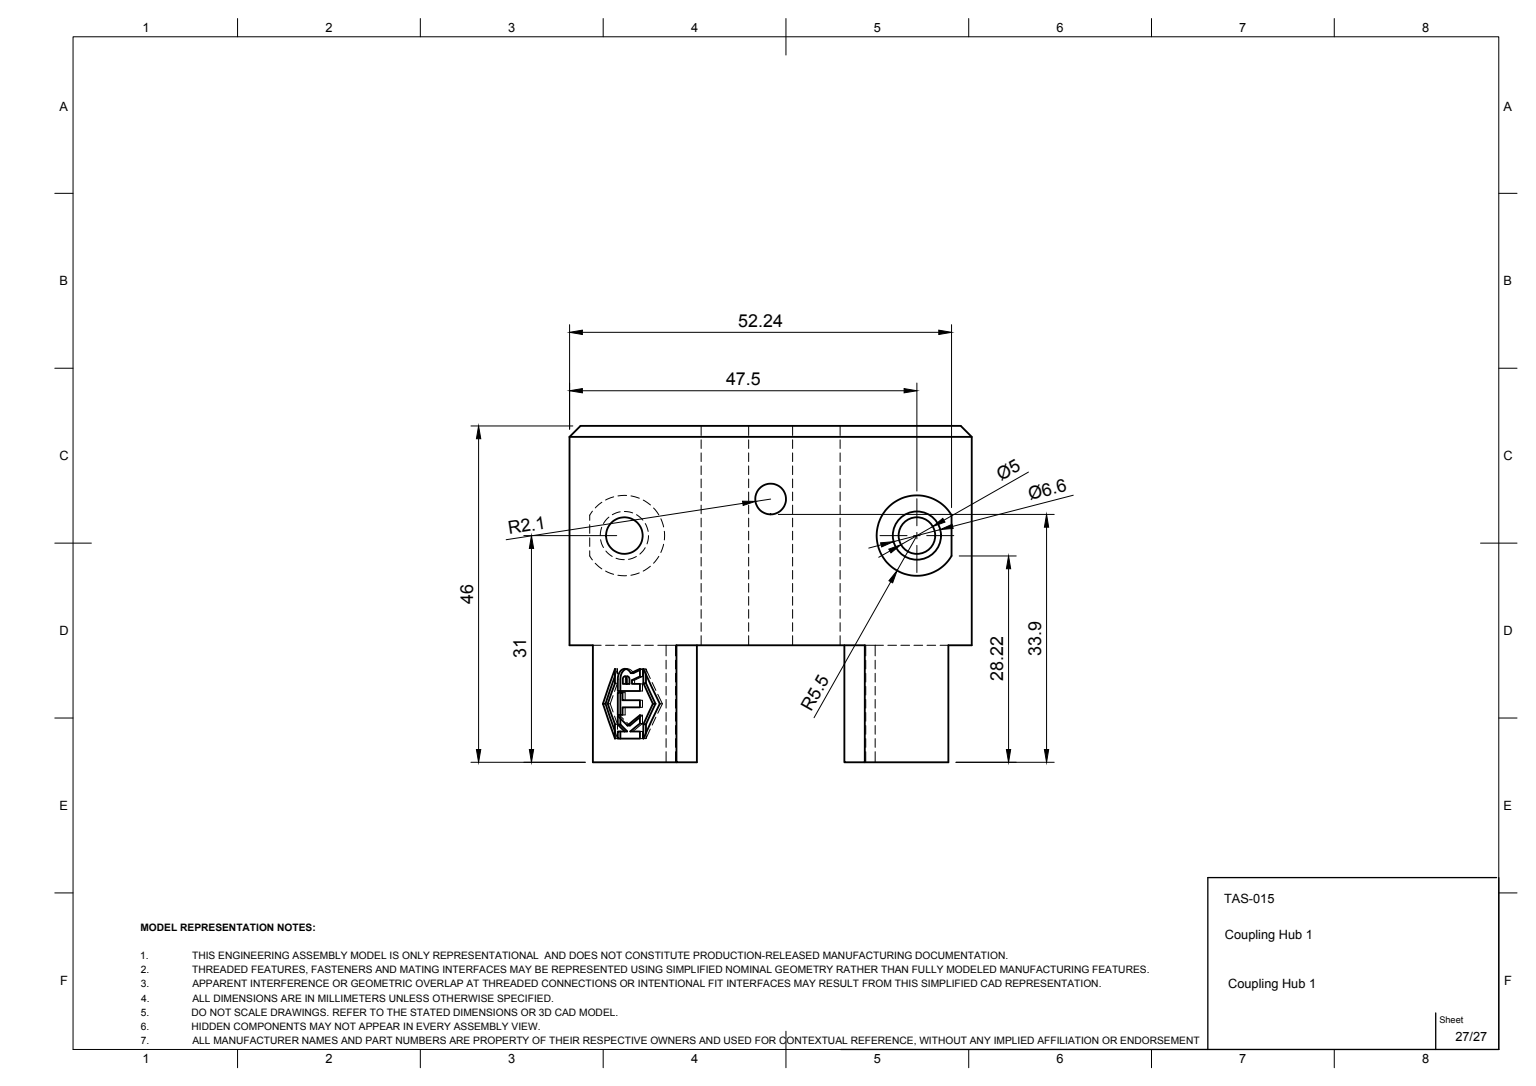
ISO-10303-21;
HEADER;
/* Generated by software containing ST-Developer
 * from STEP Tools, Inc. (www.steptools.com) 
 */

FILE_DESCRIPTION(
/* description */ ('STEP AP214'),
/* implementation_level */ '2;1');

FILE_NAME(
/* name */ 'Coupling Hub 1.step',
/* time_stamp */ '2026-11-15T14:49:54-08:00',
/* author */ (''),
/* organization */ (''),
/* preprocessor_version */ 'ST-DEVELOPER v20.2',
/* originating_system */ 'Autodesk Translation Framework v15.17.0.0',
/* authorisation */ '');

FILE_SCHEMA (('AUTOMOTIVE_DESIGN { 1 0 10303 214 3 1 1 }'));
ENDSEC;

DATA;
#10=MECHANICAL_DESIGN_GEOMETRIC_PRESENTATION_REPRESENTATION('',(#1124,#1125),#66721);
#389=B_SPLINE_CURVE_WITH_KNOTS('',3,(#65265,#65266,#65267,#65268,#65269,
#65270,#65271,#65272,#65273,#65274,#65275,#65276,#65277,#65278,#65279,#65280,
#65281,#65282),.UNSPECIFIED.,.F.,.F.,(4,2,2,2,2,2,2,2,4),(0.567634871261072,
0.624046753013484,0.757510403489333,0.849653931020164,0.941797458550995,
1.03394098608183,1.12608451361266,1.25954816408851,1.39301181456436),
 .UNSPECIFIED.);
#390=B_SPLINE_CURVE_WITH_KNOTS('',3,(#65283,#65284,#65285,#65286,#65287,
#65288,#65289,#65290,#65291,#65292,#65293,#65294,#65295,#65296,#65297,#65298,
#65299,#65300,#65301,#65302,#65303,#65304,#65305,#65306,#65307),
 .UNSPECIFIED.,.F.,.F.,(4,2,2,2,2,3,2,2,2,2,2,4),(1.39301181456436,1.54288207354147,
1.69275233251858,1.78817362481028,1.83588427095614,1.88359491710199,1.93130556324784,
1.97901620939369,2.0744375016854,2.22430776066251,2.37417801963962,2.45122978836306),
 .UNSPECIFIED.);
#391=B_SPLINE_CURVE_WITH_KNOTS('',3,(#65311,#65312,#65313,#65314,#65315,
#65316,#65317,#65318,#65319,#65320,#65321,#65322,#65323,#65324,#65325,#65326,
#65327,#65328,#65329,#65330,#65331,#65332,#65333,#65334,#65335,#65336,#65337,
#65338,#65339,#65340),.UNSPECIFIED.,.F.,.F.,(4,2,2,2,2,2,2,2,2,2,2,2,2,
2,4),(-3.98325608641923,-3.86919217466994,-3.49972652064847,-3.130260866627,
-2.85088285941104,-2.57150485219509,-2.36940240570498,-2.16729995921487,
-1.96519751272476,-1.76309506623465,-1.4837170590187,-1.20433905180275,
-0.834873397781281,-0.465407743759808,-0.351343832010516),.UNSPECIFIED.);
#392=B_SPLINE_CURVE_WITH_KNOTS('',3,(#65376,#65377,#65378,#65379,#65380,
#65381,#65382,#65383,#65384,#65385,#65386,#65387,#65388,#65389,#65390,#65391,
#65392,#65393,#65394,#65395,#65396,#65397,#65398,#65399,#65400,#65401,#65402,
#65403,#65404,#65405),.UNSPECIFIED.,.F.,.F.,(4,2,2,2,2,2,2,2,2,2,2,2,2,
2,4),(-3.98325608641923,-3.86919217466994,-3.49972652064847,-3.130260866627,
-2.85088285941104,-2.57150485219509,-2.36940240570498,-2.16729995921487,
-1.96519751272476,-1.76309506623465,-1.4837170590187,-1.20433905180275,
-0.834873397781281,-0.465407743759808,-0.351343832010517),.UNSPECIFIED.);
#393=B_SPLINE_CURVE_WITH_KNOTS('',3,(#65422,#65423,#65424,#65425,#65426,
#65427,#65428,#65429,#65430,#65431,#65432,#65433,#65434,#65435,#65436,#65437,
#65438,#65439,#65440,#65441,#65442,#65443,#65444,#65445,#65446,#65447,#65448,
#65449),.UNSPECIFIED.,.F.,.F.,(4,2,2,2,2,2,2,2,2,2,2,2,2,4),(0.490583102537635,
0.624046753013484,0.757510403489333,0.849653931020164,0.941797458550995,
1.03394098608183,1.12608451361266,1.25954816408851,1.39301181456436,1.54288207354147,
1.69275233251858,1.78817362481028,1.83588427095614,1.88359491710199),
 .UNSPECIFIED.);
#394=B_SPLINE_CURVE_WITH_KNOTS('',3,(#65450,#65451,#65452,#65453,#65454,
#65455,#65456,#65457,#65458,#65459,#65460,#65461),.UNSPECIFIED.,.F.,.F.,
(4,2,2,2,2,4),(0.,0.0477106461458525,0.095421292291705,0.19084258458341,
0.340712843560522,0.490583102537635),.UNSPECIFIED.);
#395=B_SPLINE_CURVE_WITH_KNOTS('',3,(#65538,#65539,#65540,#65541,#65542,
#65543,#65544,#65545,#65546,#65547,#65548,#65549,#65550,#65551,#65552,#65553,
#65554,#65555),.UNSPECIFIED.,.F.,.F.,(4,2,2,2,2,2,2,2,4),(0.,0.0151927838523538,
0.0303855677047076,0.0455818431537581,0.0607781186028085,0.0759788205112385,
0.0911795224196684,0.106372746681134,0.1215659709426),.UNSPECIFIED.);
#396=B_SPLINE_CURVE_WITH_KNOTS('',3,(#65565,#65566,#65567,#65568,#65569,
#65570,#65571,#65572,#65573,#65574,#65575,#65576,#65577,#65578,#65579,#65580,
#65581,#65582),.UNSPECIFIED.,.F.,.F.,(4,2,2,2,2,2,2,2,4),(0.316549052084077,
0.395686269484847,0.474823486885617,0.553960795526886,0.633098104168155,
0.712235412809424,0.791372721450693,0.870509938851463,0.949647156252233),
 .UNSPECIFIED.);
#397=B_SPLINE_CURVE_WITH_KNOTS('',3,(#65584,#65585,#65586,#65587,#65588,
#65589,#65590,#65591,#65592,#65593,#65594,#65595,#65596,#65597,#65598,#65599,
#65600,#65601,#65602,#65603,#65604,#65605,#65606,#65607,#65608,#65609,#65610,
#65611,#65612,#65613,#65614,#65615,#65616,#65617,#65618,#65619,#65620,#65621,
#65622,#65623,#65624,#65625,#65626,#65627,#65628,#65629,#65630,#65631,#65632,
#65633,#65634,#65635,#65636,#65637,#65638,#65639,#65640,#65641,#65642,#65643,
#65644),.UNSPECIFIED.,.F.,.F.,(4,3,3,3,3,3,3,3,3,3,3,3,3,3,3,3,3,3,3,3,
4),(0.,0.0530381007183943,0.106881831871485,0.160741064784848,0.214029096098922,
0.25,0.302729149593727,0.356241664754916,0.409762787712598,0.462708186143729,
0.5,0.552255845606725,0.605282211731377,0.658318725202785,0.710788396890028,
0.75,0.802421738286123,0.855626872467919,0.908846463729713,0.961502691971665,
1.),.UNSPECIFIED.);
#398=B_SPLINE_CURVE_WITH_KNOTS('',3,(#65645,#65646,#65647,#65648,#65649,
#65650,#65651,#65652,#65653,#65654),.UNSPECIFIED.,.F.,.F.,(4,2,2,2,4),(0.949647156252233,
1.028784373653,1.10792159105377,1.18705889969504,1.26619620833631),
 .UNSPECIFIED.);
#399=B_SPLINE_CURVE_WITH_KNOTS('',3,(#65695,#65696,#65697,#65698,#65699,
#65700,#65701,#65702,#65703,#65704,#65705,#65706,#65707,#65708,#65709,#65710),
 .UNSPECIFIED.,.F.,.F.,(4,2,2,2,2,2,2,4),(-0.779703847201593,-0.757646703299412,
-0.7035492015768,-0.649451699854188,-0.595298023055894,-0.5411443462576,
-0.487035463795603,-0.432926581333605),.UNSPECIFIED.);
#400=B_SPLINE_CURVE_WITH_KNOTS('',3,(#65933,#65934,#65935,#65936,#65937,
#65938,#65939,#65940,#65941,#65942,#65943,#65944,#65945,#65946,#65947,#65948),
 .UNSPECIFIED.,.F.,.F.,(4,2,2,2,2,2,2,4),(0.432932407296797,0.487041759940904,
0.541151112585012,0.595306935250484,0.649462757915956,0.703560301016107,
0.757657844116259,0.779715370662845),.UNSPECIFIED.);
#401=B_SPLINE_CURVE_WITH_KNOTS('',3,(#65980,#65981,#65982,#65983,#65984,
#65985,#65986,#65987,#65988,#65989,#65990,#65991,#65992,#65993,#65994,#65995,
#65996,#65997),.UNSPECIFIED.,.F.,.F.,(4,2,2,2,2,2,2,2,4),(0.121566783856533,
0.136760015420318,0.151953246984103,0.167154235901664,0.182355224819225,
0.197551621622939,0.212748018426654,0.22794079306986,0.243133567713066),
 .UNSPECIFIED.);
#557=CONICAL_SURFACE('',#28270,26.75,0.785398163397448);
#558=CONICAL_SURFACE('',#28333,26.75,0.785398163397448);
#679=ELLIPSE('',#28381,55.0000000336669,27.5000000339144);
#680=ELLIPSE('',#28382,55.0000002451225,27.5000002404132);
#681=ELLIPSE('',#28383,54.9999999054554,27.4999999087398);
#682=ELLIPSE('',#28384,54.9999999692227,27.4999999704721);
#683=ELLIPSE('',#28385,32.156845610475,27.5);
#684=ELLIPSE('',#28391,33.1709935839343,27.5);
#685=ELLIPSE('',#28392,55.0000000340055,27.5000000342412);
#686=ELLIPSE('',#28393,54.9999999479979,27.4999999499152);
#687=ELLIPSE('',#28394,54.99999995367,27.4999999554067);
#688=ELLIPSE('',#28395,55.0000002756688,27.5000002701183);
#689=ELLIPSE('',#28410,31.5721756903194,27.);
#690=ELLIPSE('',#28413,31.5721756902845,27.);
#691=ELLIPSE('',#28426,32.5678846096809,27.);
#692=ELLIPSE('',#28429,54.0000000112232,27.0000000109264);
#693=ELLIPSE('',#28430,54.00000012479,27.0000001227984);
#694=ELLIPSE('',#28431,53.999999886139,26.9999998900941);
#695=ELLIPSE('',#28432,53.9999999927924,26.9999999931258);
#696=ELLIPSE('',#28441,53.9999999968904,26.9999999970926);
#697=ELLIPSE('',#28443,53.9999999996556,26.9999999997697);
#698=ELLIPSE('',#28446,53.9999999562436,26.9999999583659);
#699=ELLIPSE('',#28448,53.9999995905245,26.999999602125);
#1061=SHAPE_REPRESENTATION_RELATIONSHIP('SRR','None',#66924,#1092);
#1092=ADVANCED_BREP_SHAPE_REPRESENTATION('',(#1159,#1160),#66715);
#1124=STYLED_ITEM('',(#67095),#1159);
#1125=STYLED_ITEM('',(#67095),#1160);
#1159=MANIFOLD_SOLID_BREP('Body1',#25690);
#1160=MANIFOLD_SOLID_BREP('Body2',#25691);
#1432=FACE_BOUND('',#5208,.T.);
#1433=FACE_BOUND('',#5209,.T.);
#1434=FACE_BOUND('',#5214,.T.);
#1435=FACE_BOUND('',#5217,.T.);
#1436=FACE_BOUND('',#5220,.T.);
#1437=FACE_BOUND('',#5222,.T.);
#1438=FACE_BOUND('',#5226,.T.);
#1439=FACE_BOUND('',#5230,.T.);
#1440=FACE_BOUND('',#5233,.T.);
#1441=FACE_BOUND('',#5235,.T.);
#1442=FACE_BOUND('',#5246,.T.);
#1443=FACE_BOUND('',#5256,.T.);
#1444=FACE_BOUND('',#5257,.T.);
#1445=FACE_BOUND('',#5258,.T.);
#1446=FACE_BOUND('',#5259,.T.);
#1447=FACE_BOUND('',#5260,.T.);
#1448=FACE_BOUND('',#5261,.T.);
#1449=FACE_BOUND('',#5262,.T.);
#1450=FACE_BOUND('',#5263,.T.);
#1451=FACE_BOUND('',#5313,.T.);
#2148=PLANE('',#28267);
#2149=PLANE('',#28272);
#2150=PLANE('',#28277);
#2151=PLANE('',#28300);
#2152=PLANE('',#28303);
#2153=PLANE('',#28308);
#2154=PLANE('',#28312);
#2155=PLANE('',#28313);
#2156=PLANE('',#28317);
#2157=PLANE('',#28323);
#2158=PLANE('',#28327);
#2159=PLANE('',#28328);
#2160=PLANE('',#28329);
#2161=PLANE('',#28335);
#2162=PLANE('',#28353);
#2163=PLANE('',#28354);
#2164=PLANE('',#28355);
#2165=PLANE('',#28368);
#2166=PLANE('',#28370);
#2167=PLANE('',#28401);
#2168=PLANE('',#28402);
#2169=PLANE('',#28403);
#2170=PLANE('',#28404);
#2171=PLANE('',#28405);
#2172=PLANE('',#28406);
#2173=PLANE('',#28407);
#2174=PLANE('',#28408);
#2175=PLANE('',#28409);
#2176=PLANE('',#28411);
#2177=PLANE('',#28412);
#2178=PLANE('',#28414);
#2179=PLANE('',#28415);
#2180=PLANE('',#28417);
#2181=PLANE('',#28419);
#2182=PLANE('',#28420);
#2183=PLANE('',#28422);
#2184=PLANE('',#28423);
#2185=PLANE('',#28425);
#2186=PLANE('',#28433);
#2187=PLANE('',#28434);
#2188=PLANE('',#28435);
#2189=PLANE('',#28436);
#2190=PLANE('',#28437);
#2191=PLANE('',#28438);
#2192=PLANE('',#28439);
#2193=PLANE('',#28440);
#2194=PLANE('',#28442);
#2195=PLANE('',#28444);
#2196=PLANE('',#28445);
#2197=PLANE('',#28447);
#2198=PLANE('',#28450);
#2199=PLANE('',#28452);
#2200=PLANE('',#28453);
#2201=PLANE('',#28456);
#2202=PLANE('',#28457);
#2203=PLANE('',#28459);
#2204=PLANE('',#28460);
#2205=PLANE('',#28462);
#2206=PLANE('',#28463);
#2207=PLANE('',#28465);
#2208=PLANE('',#28467);
#3491=FACE_OUTER_BOUND('',#5197,.T.);
#3492=FACE_OUTER_BOUND('',#5198,.T.);
#3493=FACE_OUTER_BOUND('',#5199,.T.);
#3494=FACE_OUTER_BOUND('',#5200,.T.);
#3495=FACE_OUTER_BOUND('',#5201,.T.);
#3496=FACE_OUTER_BOUND('',#5202,.T.);
#3497=FACE_OUTER_BOUND('',#5203,.T.);
#3498=FACE_OUTER_BOUND('',#5204,.T.);
#3499=FACE_OUTER_BOUND('',#5205,.T.);
#3500=FACE_OUTER_BOUND('',#5206,.T.);
#3501=FACE_OUTER_BOUND('',#5207,.T.);
#3502=FACE_OUTER_BOUND('',#5210,.T.);
#3503=FACE_OUTER_BOUND('',#5211,.T.);
#3504=FACE_OUTER_BOUND('',#5212,.T.);
#3505=FACE_OUTER_BOUND('',#5213,.T.);
#3506=FACE_OUTER_BOUND('',#5215,.T.);
#3507=FACE_OUTER_BOUND('',#5216,.T.);
#3508=FACE_OUTER_BOUND('',#5218,.T.);
#3509=FACE_OUTER_BOUND('',#5219,.T.);
#3510=FACE_OUTER_BOUND('',#5221,.T.);
#3511=FACE_OUTER_BOUND('',#5223,.T.);
#3512=FACE_OUTER_BOUND('',#5224,.T.);
#3513=FACE_OUTER_BOUND('',#5225,.T.);
#3514=FACE_OUTER_BOUND('',#5227,.T.);
#3515=FACE_OUTER_BOUND('',#5228,.T.);
#3516=FACE_OUTER_BOUND('',#5229,.T.);
#3517=FACE_OUTER_BOUND('',#5231,.T.);
#3518=FACE_OUTER_BOUND('',#5232,.T.);
#3519=FACE_OUTER_BOUND('',#5234,.T.);
#3520=FACE_OUTER_BOUND('',#5236,.T.);
#3521=FACE_OUTER_BOUND('',#5237,.T.);
#3522=FACE_OUTER_BOUND('',#5238,.T.);
#3523=FACE_OUTER_BOUND('',#5239,.T.);
#3524=FACE_OUTER_BOUND('',#5240,.T.);
#3525=FACE_OUTER_BOUND('',#5241,.T.);
#3526=FACE_OUTER_BOUND('',#5242,.T.);
#3527=FACE_OUTER_BOUND('',#5243,.T.);
#3528=FACE_OUTER_BOUND('',#5244,.T.);
#3529=FACE_OUTER_BOUND('',#5245,.T.);
#3530=FACE_OUTER_BOUND('',#5247,.T.);
#3531=FACE_OUTER_BOUND('',#5248,.T.);
#3532=FACE_OUTER_BOUND('',#5249,.T.);
#3533=FACE_OUTER_BOUND('',#5250,.T.);
#3534=FACE_OUTER_BOUND('',#5251,.T.);
#3535=FACE_OUTER_BOUND('',#5252,.T.);
#3536=FACE_OUTER_BOUND('',#5253,.T.);
#3537=FACE_OUTER_BOUND('',#5254,.T.);
#3538=FACE_OUTER_BOUND('',#5255,.T.);
#3539=FACE_OUTER_BOUND('',#5264,.T.);
#3540=FACE_OUTER_BOUND('',#5265,.T.);
#3541=FACE_OUTER_BOUND('',#5266,.T.);
#3542=FACE_OUTER_BOUND('',#5267,.T.);
#3543=FACE_OUTER_BOUND('',#5268,.T.);
#3544=FACE_OUTER_BOUND('',#5269,.T.);
#3545=FACE_OUTER_BOUND('',#5270,.T.);
#3546=FACE_OUTER_BOUND('',#5271,.T.);
#3547=FACE_OUTER_BOUND('',#5272,.T.);
#3548=FACE_OUTER_BOUND('',#5273,.T.);
#3549=FACE_OUTER_BOUND('',#5274,.T.);
#3550=FACE_OUTER_BOUND('',#5275,.T.);
#3551=FACE_OUTER_BOUND('',#5276,.T.);
#3552=FACE_OUTER_BOUND('',#5277,.T.);
#3553=FACE_OUTER_BOUND('',#5278,.T.);
#3554=FACE_OUTER_BOUND('',#5279,.T.);
#3555=FACE_OUTER_BOUND('',#5280,.T.);
#3556=FACE_OUTER_BOUND('',#5281,.T.);
#3557=FACE_OUTER_BOUND('',#5282,.T.);
#3558=FACE_OUTER_BOUND('',#5283,.T.);
#3559=FACE_OUTER_BOUND('',#5284,.T.);
#3560=FACE_OUTER_BOUND('',#5285,.T.);
#3561=FACE_OUTER_BOUND('',#5286,.T.);
#3562=FACE_OUTER_BOUND('',#5287,.T.);
#3563=FACE_OUTER_BOUND('',#5288,.T.);
#3564=FACE_OUTER_BOUND('',#5289,.T.);
#3565=FACE_OUTER_BOUND('',#5290,.T.);
#3566=FACE_OUTER_BOUND('',#5291,.T.);
#3567=FACE_OUTER_BOUND('',#5292,.T.);
#3568=FACE_OUTER_BOUND('',#5293,.T.);
#3569=FACE_OUTER_BOUND('',#5294,.T.);
#3570=FACE_OUTER_BOUND('',#5295,.T.);
#3571=FACE_OUTER_BOUND('',#5296,.T.);
#3572=FACE_OUTER_BOUND('',#5297,.T.);
#3573=FACE_OUTER_BOUND('',#5298,.T.);
#3574=FACE_OUTER_BOUND('',#5299,.T.);
#3575=FACE_OUTER_BOUND('',#5300,.T.);
#3576=FACE_OUTER_BOUND('',#5301,.T.);
#3577=FACE_OUTER_BOUND('',#5302,.T.);
#3578=FACE_OUTER_BOUND('',#5303,.T.);
#3579=FACE_OUTER_BOUND('',#5304,.T.);
#3580=FACE_OUTER_BOUND('',#5305,.T.);
#3581=FACE_OUTER_BOUND('',#5306,.T.);
#3582=FACE_OUTER_BOUND('',#5307,.T.);
#3583=FACE_OUTER_BOUND('',#5308,.T.);
#3584=FACE_OUTER_BOUND('',#5309,.T.);
#3585=FACE_OUTER_BOUND('',#5310,.T.);
#3586=FACE_OUTER_BOUND('',#5311,.T.);
#3587=FACE_OUTER_BOUND('',#5312,.T.);
#5197=EDGE_LOOP('',(#22764,#22765,#22766,#22767));
#5198=EDGE_LOOP('',(#22768,#22769,#22770,#22771));
#5199=EDGE_LOOP('',(#22772,#22773,#22774,#22775));
#5200=EDGE_LOOP('',(#22776,#22777,#22778,#22779));
#5201=EDGE_LOOP('',(#22780,#22781,#22782,#22783));
#5202=EDGE_LOOP('',(#22784,#22785,#22786,#22787));
#5203=EDGE_LOOP('',(#22788,#22789,#22790,#22791));
#5204=EDGE_LOOP('',(#22792,#22793,#22794,#22795));
#5205=EDGE_LOOP('',(#22796,#22797,#22798,#22799));
#5206=EDGE_LOOP('',(#22800,#22801,#22802,#22803));
#5207=EDGE_LOOP('',(#22804,#22805,#22806,#22807,#22808,#22809,#22810,#22811,
#22812,#22813,#22814,#22815));
#5208=EDGE_LOOP('',(#22816,#22817));
#5209=EDGE_LOOP('',(#22818,#22819));
#5210=EDGE_LOOP('',(#22820,#22821,#22822,#22823));
#5211=EDGE_LOOP('',(#22824,#22825,#22826,#22827,#22828,#22829,#22830,#22831,
#22832,#22833,#22834,#22835));
#5212=EDGE_LOOP('',(#22836,#22837,#22838,#22839,#22840));
#5213=EDGE_LOOP('',(#22841,#22842));
#5214=EDGE_LOOP('',(#22843));
#5215=EDGE_LOOP('',(#22844,#22845,#22846,#22847));
#5216=EDGE_LOOP('',(#22848));
#5217=EDGE_LOOP('',(#22849));
#5218=EDGE_LOOP('',(#22850,#22851,#22852,#22853));
#5219=EDGE_LOOP('',(#22854,#22855,#22856,#22857,#22858));
#5220=EDGE_LOOP('',(#22859));
#5221=EDGE_LOOP('',(#22860,#22861,#22862,#22863,#22864));
#5222=EDGE_LOOP('',(#22865));
#5223=EDGE_LOOP('',(#22866,#22867));
#5224=EDGE_LOOP('',(#22868,#22869));
#5225=EDGE_LOOP('',(#22870,#22871,#22872,#22873,#22874));
#5226=EDGE_LOOP('',(#22875));
#5227=EDGE_LOOP('',(#22876,#22877,#22878,#22879,#22880));
#5228=EDGE_LOOP('',(#22881,#22882,#22883,#22884));
#5229=EDGE_LOOP('',(#22885));
#5230=EDGE_LOOP('',(#22886));
#5231=EDGE_LOOP('',(#22887,#22888,#22889,#22890));
#5232=EDGE_LOOP('',(#22891,#22892));
#5233=EDGE_LOOP('',(#22893));
#5234=EDGE_LOOP('',(#22894,#22895,#22896,#22897,#22898));
#5235=EDGE_LOOP('',(#22899));
#5236=EDGE_LOOP('',(#22900,#22901,#22902,#22903,#22904,#22905,#22906,#22907));
#5237=EDGE_LOOP('',(#22908,#22909,#22910,#22911));
#5238=EDGE_LOOP('',(#22912,#22913,#22914,#22915,#22916,#22917,#22918,#22919,
#22920,#22921,#22922,#22923,#22924,#22925,#22926,#22927));
#5239=EDGE_LOOP('',(#22928,#22929,#22930,#22931));
#5240=EDGE_LOOP('',(#22932,#22933,#22934,#22935));
#5241=EDGE_LOOP('',(#22936,#22937,#22938,#22939));
#5242=EDGE_LOOP('',(#22940,#22941,#22942,#22943,#22944,#22945));
#5243=EDGE_LOOP('',(#22946,#22947,#22948,#22949));
#5244=EDGE_LOOP('',(#22950,#22951,#22952,#22953));
#5245=EDGE_LOOP('',(#22954,#22955,#22956,#22957));
#5246=EDGE_LOOP('',(#22958));
#5247=EDGE_LOOP('',(#22959,#22960,#22961,#22962));
#5248=EDGE_LOOP('',(#22963,#22964,#22965,#22966));
#5249=EDGE_LOOP('',(#22967,#22968,#22969,#22970));
#5250=EDGE_LOOP('',(#22971,#22972,#22973,#22974));
#5251=EDGE_LOOP('',(#22975,#22976,#22977,#22978));
#5252=EDGE_LOOP('',(#22979,#22980,#22981,#22982));
#5253=EDGE_LOOP('',(#22983,#22984,#22985,#22986));
#5254=EDGE_LOOP('',(#22987,#22988,#22989,#22990));
#5255=EDGE_LOOP('',(#22991,#22992,#22993,#22994,#22995,#22996,#22997,#22998,
#22999,#23000,#23001,#23002));
#5256=EDGE_LOOP('',(#23003,#23004));
#5257=EDGE_LOOP('',(#23005,#23006,#23007,#23008,#23009,#23010,#23011,#23012,
#23013));
#5258=EDGE_LOOP('',(#23014,#23015,#23016,#23017,#23018,#23019,#23020,#23021));
#5259=EDGE_LOOP('',(#23022,#23023,#23024));
#5260=EDGE_LOOP('',(#23025,#23026));
#5261=EDGE_LOOP('',(#23027,#23028,#23029,#23030,#23031,#23032));
#5262=EDGE_LOOP('',(#23033,#23034,#23035,#23036,#23037,#23038,#23039,#23040,
#23041,#23042,#23043));
#5263=EDGE_LOOP('',(#23044,#23045,#23046,#23047,#23048,#23049));
#5264=EDGE_LOOP('',(#23050,#23051,#23052,#23053,#23054,#23055,#23056,#23057));
#5265=EDGE_LOOP('',(#23058,#23059,#23060,#23061));
#5266=EDGE_LOOP('',(#23062,#23063,#23064,#23065));
#5267=EDGE_LOOP('',(#23066,#23067,#23068,#23069));
#5268=EDGE_LOOP('',(#23070,#23071,#23072,#23073));
#5269=EDGE_LOOP('',(#23074,#23075,#23076,#23077));
#5270=EDGE_LOOP('',(#23078,#23079,#23080,#23081));
#5271=EDGE_LOOP('',(#23082,#23083,#23084,#23085));
#5272=EDGE_LOOP('',(#23086,#23087,#23088,#23089));
#5273=EDGE_LOOP('',(#23090,#23091,#23092,#23093));
#5274=EDGE_LOOP('',(#23094,#23095,#23096,#23097));
#5275=EDGE_LOOP('',(#23098,#23099,#23100,#23101));
#5276=EDGE_LOOP('',(#23102,#23103,#23104,#23105));
#5277=EDGE_LOOP('',(#23106,#23107,#23108,#23109));
#5278=EDGE_LOOP('',(#23110,#23111,#23112,#23113));
#5279=EDGE_LOOP('',(#23114,#23115,#23116,#23117));
#5280=EDGE_LOOP('',(#23118,#23119,#23120,#23121));
#5281=EDGE_LOOP('',(#23122,#23123,#23124,#23125));
#5282=EDGE_LOOP('',(#23126,#23127,#23128,#23129));
#5283=EDGE_LOOP('',(#23130,#23131,#23132,#23133));
#5284=EDGE_LOOP('',(#23134,#23135,#23136,#23137,#23138,#23139,#23140,#23141,
#23142,#23143,#23144));
#5285=EDGE_LOOP('',(#23145,#23146,#23147,#23148,#23149,#23150));
#5286=EDGE_LOOP('',(#23151,#23152,#23153,#23154));
#5287=EDGE_LOOP('',(#23155,#23156,#23157,#23158));
#5288=EDGE_LOOP('',(#23159,#23160,#23161,#23162));
#5289=EDGE_LOOP('',(#23163,#23164,#23165,#23166));
#5290=EDGE_LOOP('',(#23167,#23168,#23169,#23170));
#5291=EDGE_LOOP('',(#23171,#23172,#23173,#23174));
#5292=EDGE_LOOP('',(#23175,#23176,#23177,#23178));
#5293=EDGE_LOOP('',(#23179,#23180,#23181,#23182));
#5294=EDGE_LOOP('',(#23183,#23184,#23185,#23186));
#5295=EDGE_LOOP('',(#23187,#23188,#23189,#23190));
#5296=EDGE_LOOP('',(#23191,#23192,#23193,#23194));
#5297=EDGE_LOOP('',(#23195,#23196,#23197,#23198));
#5298=EDGE_LOOP('',(#23199,#23200,#23201,#23202,#23203,#23204));
#5299=EDGE_LOOP('',(#23205,#23206,#23207,#23208));
#5300=EDGE_LOOP('',(#23209,#23210,#23211,#23212));
#5301=EDGE_LOOP('',(#23213,#23214,#23215,#23216));
#5302=EDGE_LOOP('',(#23217,#23218,#23219,#23220));
#5303=EDGE_LOOP('',(#23221,#23222,#23223,#23224));
#5304=EDGE_LOOP('',(#23225,#23226,#23227,#23228));
#5305=EDGE_LOOP('',(#23229,#23230,#23231,#23232));
#5306=EDGE_LOOP('',(#23233,#23234,#23235,#23236));
#5307=EDGE_LOOP('',(#23237,#23238,#23239,#23240));
#5308=EDGE_LOOP('',(#23241,#23242,#23243,#23244));
#5309=EDGE_LOOP('',(#23245,#23246,#23247,#23248));
#5310=EDGE_LOOP('',(#23249,#23250,#23251,#23252));
#5311=EDGE_LOOP('',(#23253,#23254,#23255,#23256));
#5312=EDGE_LOOP('',(#23257,#23258,#23259,#23260,#23261,#23262,#23263,#23264,
#23265));
#5313=EDGE_LOOP('',(#23266,#23267,#23268,#23269));
#7166=LINE('',#65197,#9155);
#7167=LINE('',#65201,#9156);
#7168=LINE('',#65207,#9157);
#7169=LINE('',#65208,#9158);
#7170=LINE('',#65231,#9159);
#7171=LINE('',#65232,#9160);
#7172=LINE('',#65235,#9161);
#7173=LINE('',#65237,#9162);
#7174=LINE('',#65241,#9163);
#7175=LINE('',#65245,#9164);
#7176=LINE('',#65250,#9165);
#7177=LINE('',#65254,#9166);
#7178=LINE('',#65259,#9167);
#7179=LINE('',#65261,#9168);
#7180=LINE('',#65310,#9169);
#7181=LINE('',#65343,#9170);
#7182=LINE('',#65346,#9171);
#7183=LINE('',#65348,#9172);
#7184=LINE('',#65349,#9173);
#7185=LINE('',#65352,#9174);
#7186=LINE('',#65361,#9175);
#7187=LINE('',#65368,#9176);
#7188=LINE('',#65409,#9177);
#7189=LINE('',#65411,#9178);
#7190=LINE('',#65413,#9179);
#7191=LINE('',#65415,#9180);
#7192=LINE('',#65416,#9181);
#7193=LINE('',#65462,#9182);
#7194=LINE('',#65467,#9183);
#7195=LINE('',#65474,#9184);
#7196=LINE('',#65477,#9185);
#7197=LINE('',#65481,#9186);
#7198=LINE('',#65483,#9187);
#7199=LINE('',#65485,#9188);
#7200=LINE('',#65487,#9189);
#7201=LINE('',#65488,#9190);
#7202=LINE('',#65493,#9191);
#7203=LINE('',#65495,#9192);
#7204=LINE('',#65497,#9193);
#7205=LINE('',#65523,#9194);
#7206=LINE('',#65525,#9195);
#7207=LINE('',#65527,#9196);
#7208=LINE('',#65530,#9197);
#7209=LINE('',#65532,#9198);
#7210=LINE('',#65536,#9199);
#7211=LINE('',#65557,#9200);
#7212=LINE('',#65563,#9201);
#7213=LINE('',#65656,#9202);
#7214=LINE('',#65658,#9203);
#7215=LINE('',#65664,#9204);
#7216=LINE('',#65665,#9205);
#7217=LINE('',#65670,#9206);
#7218=LINE('',#65671,#9207);
#7219=LINE('',#65674,#9208);
#7220=LINE('',#65677,#9209);
#7221=LINE('',#65681,#9210);
#7222=LINE('',#65686,#9211);
#7223=LINE('',#65714,#9212);
#7224=LINE('',#65718,#9213);
#7225=LINE('',#65722,#9214);
#7226=LINE('',#65725,#9215);
#7227=LINE('',#65730,#9216);
#7228=LINE('',#65734,#9217);
#7229=LINE('',#65738,#9218);
#7230=LINE('',#65741,#9219);
#7231=LINE('',#65744,#9220);
#7232=LINE('',#65750,#9221);
#7233=LINE('',#65758,#9222);
#7234=LINE('',#65764,#9223);
#7235=LINE('',#65768,#9224);
#7236=LINE('',#65774,#9225);
#7237=LINE('',#65780,#9226);
#7238=LINE('',#65786,#9227);
#7239=LINE('',#65793,#9228);
#7240=LINE('',#65797,#9229);
#7241=LINE('',#65801,#9230);
#7242=LINE('',#65804,#9231);
#7243=LINE('',#65806,#9232);
#7244=LINE('',#65807,#9233);
#7245=LINE('',#65809,#9234);
#7246=LINE('',#65811,#9235);
#7247=LINE('',#65813,#9236);
#7248=LINE('',#65815,#9237);
#7249=LINE('',#65817,#9238);
#7250=LINE('',#65819,#9239);
#7251=LINE('',#65823,#9240);
#7252=LINE('',#65826,#9241);
#7253=LINE('',#65829,#9242);
#7254=LINE('',#65830,#9243);
#7255=LINE('',#65833,#9244);
#7256=LINE('',#65837,#9245);
#7257=LINE('',#65839,#9246);
#7258=LINE('',#65840,#9247);
#7259=LINE('',#65843,#9248);
#7260=LINE('',#65847,#9249);
#7261=LINE('',#65851,#9250);
#7262=LINE('',#65852,#9251);
#7263=LINE('',#65855,#9252);
#7264=LINE('',#65859,#9253);
#7265=LINE('',#65860,#9254);
#7266=LINE('',#65871,#9255);
#7267=LINE('',#65877,#9256);
#7268=LINE('',#65880,#9257);
#7269=LINE('',#65881,#9258);
#7270=LINE('',#65883,#9259);
#7271=LINE('',#65885,#9260);
#7272=LINE('',#65887,#9261);
#7273=LINE('',#65889,#9262);
#7274=LINE('',#65893,#9263);
#7275=LINE('',#65895,#9264);
#7276=LINE('',#65896,#9265);
#7277=LINE('',#65899,#9266);
#7278=LINE('',#65903,#9267);
#7279=LINE('',#65907,#9268);
#7280=LINE('',#65908,#9269);
#7281=LINE('',#65912,#9270);
#7282=LINE('',#65918,#9271);
#7283=LINE('',#65921,#9272);
#7284=LINE('',#65924,#9273);
#7285=LINE('',#65925,#9274);
#7286=LINE('',#65928,#9275);
#7287=LINE('',#65932,#9276);
#7288=LINE('',#65951,#9277);
#7289=LINE('',#65952,#9278);
#7290=LINE('',#65955,#9279);
#7291=LINE('',#65958,#9280);
#7292=LINE('',#65961,#9281);
#7293=LINE('',#65962,#9282);
#7294=LINE('',#65965,#9283);
#7295=LINE('',#65969,#9284);
#7296=LINE('',#65970,#9285);
#7297=LINE('',#65973,#9286);
#7298=LINE('',#65976,#9287);
#7299=LINE('',#65979,#9288);
#7300=LINE('',#65999,#9289);
#9155=VECTOR('',#34893,1000.);
#9156=VECTOR('',#34896,1000.);
#9157=VECTOR('',#34903,1000.);
#9158=VECTOR('',#34904,1000.);
#9159=VECTOR('',#34929,1000.);
#9160=VECTOR('',#34930,1000.);
#9161=VECTOR('',#34933,1000.);
#9162=VECTOR('',#34934,1000.);
#9163=VECTOR('',#34939,1000.);
#9164=VECTOR('',#34944,1000.);
#9165=VECTOR('',#34951,1000.);
#9166=VECTOR('',#34956,1000.);
#9167=VECTOR('',#34963,1000.);
#9168=VECTOR('',#34964,1000.);
#9169=VECTOR('',#34967,1000.);
#9170=VECTOR('',#34970,1000.);
#9171=VECTOR('',#34973,1000.);
#9172=VECTOR('',#34976,1000.);
#9173=VECTOR('',#34977,1000.);
#9174=VECTOR('',#34980,2.5);
#9175=VECTOR('',#34993,3.3);
#9176=VECTOR('',#35002,2.5);
#9177=VECTOR('',#35015,1000.);
#9178=VECTOR('',#35016,1000.);
#9179=VECTOR('',#35017,1000.);
#9180=VECTOR('',#35018,1000.);
#9181=VECTOR('',#35019,1000.);
#9182=VECTOR('',#35024,2.5);
#9183=VECTOR('',#35029,2.5);
#9184=VECTOR('',#35038,3.3);
#9185=VECTOR('',#35043,1000.);
#9186=VECTOR('',#35046,1000.);
#9187=VECTOR('',#35047,1000.);
#9188=VECTOR('',#35048,1000.);
#9189=VECTOR('',#35049,1000.);
#9190=VECTOR('',#35050,1000.);
#9191=VECTOR('',#35055,1000.);
#9192=VECTOR('',#35056,1000.);
#9193=VECTOR('',#35057,1000.);
#9194=VECTOR('',#35088,1000.);
#9195=VECTOR('',#35089,1000.);
#9196=VECTOR('',#35090,1000.);
#9197=VECTOR('',#35095,1000.);
#9198=VECTOR('',#35098,1000.);
#9199=VECTOR('',#35101,1000.);
#9200=VECTOR('',#35102,1000.);
#9201=VECTOR('',#35109,2.1);
#9202=VECTOR('',#35112,1000.);
#9203=VECTOR('',#35115,1000.);
#9204=VECTOR('',#35122,1000.);
#9205=VECTOR('',#35123,1000.);
#9206=VECTOR('',#35128,1000.);
#9207=VECTOR('',#35129,1000.);
#9208=VECTOR('',#35132,1000.);
#9209=VECTOR('',#35135,1000.);
#9210=VECTOR('',#35140,1000.);
#9211=VECTOR('',#35147,1000.);
#9212=VECTOR('',#35162,1000.);
#9213=VECTOR('',#35165,1000.);
#9214=VECTOR('',#35168,1000.);
#9215=VECTOR('',#35171,1000.);
#9216=VECTOR('',#35174,1000.);
#9217=VECTOR('',#35177,1000.);
#9218=VECTOR('',#35180,1000.);
#9219=VECTOR('',#35183,1000.);
#9220=VECTOR('',#35184,1000.);
#9221=VECTOR('',#35189,1000.);
#9222=VECTOR('',#35196,1000.);
#9223=VECTOR('',#35201,1000.);
#9224=VECTOR('',#35204,1000.);
#9225=VECTOR('',#35209,1000.);
#9226=VECTOR('',#35214,1000.);
#9227=VECTOR('',#35219,1000.);
#9228=VECTOR('',#35226,1000.);
#9229=VECTOR('',#35229,1000.);
#9230=VECTOR('',#35232,1000.);
#9231=VECTOR('',#35235,1000.);
#9232=VECTOR('',#35238,1000.);
#9233=VECTOR('',#35239,1000.);
#9234=VECTOR('',#35242,1000.);
#9235=VECTOR('',#35245,1000.);
#9236=VECTOR('',#35248,1000.);
#9237=VECTOR('',#35251,1000.);
#9238=VECTOR('',#35254,1000.);
#9239=VECTOR('',#35257,1000.);
#9240=VECTOR('',#35262,1000.);
#9241=VECTOR('',#35265,1000.);
#9242=VECTOR('',#35268,1000.);
#9243=VECTOR('',#35269,1000.);
#9244=VECTOR('',#35272,1000.);
#9245=VECTOR('',#35277,1000.);
#9246=VECTOR('',#35278,1000.);
#9247=VECTOR('',#35279,1000.);
#9248=VECTOR('',#35282,1000.);
#9249=VECTOR('',#35287,1000.);
#9250=VECTOR('',#35292,1000.);
#9251=VECTOR('',#35293,1000.);
#9252=VECTOR('',#35296,1000.);
#9253=VECTOR('',#35301,1000.);
#9254=VECTOR('',#35302,1000.);
#9255=VECTOR('',#35317,1000.);
#9256=VECTOR('',#35322,1000.);
#9257=VECTOR('',#35327,1000.);
#9258=VECTOR('',#35328,1000.);
#9259=VECTOR('',#35331,1000.);
#9260=VECTOR('',#35334,1000.);
#9261=VECTOR('',#35337,1000.);
#9262=VECTOR('',#35340,1000.);
#9263=VECTOR('',#35345,1000.);
#9264=VECTOR('',#35346,1000.);
#9265=VECTOR('',#35347,1000.);
#9266=VECTOR('',#35350,1000.);
#9267=VECTOR('',#35355,1000.);
#9268=VECTOR('',#35360,1000.);
#9269=VECTOR('',#35361,1000.);
#9270=VECTOR('',#35366,1000.);
#9271=VECTOR('',#35375,1000.);
#9272=VECTOR('',#35378,1000.);
#9273=VECTOR('',#35381,1000.);
#9274=VECTOR('',#35382,1000.);
#9275=VECTOR('',#35385,1000.);
#9276=VECTOR('',#35390,1000.);
#9277=VECTOR('',#35393,1000.);
#9278=VECTOR('',#35394,1000.);
#9279=VECTOR('',#35397,1000.);
#9280=VECTOR('',#35400,1000.);
#9281=VECTOR('',#35403,1000.);
#9282=VECTOR('',#35404,1000.);
#9283=VECTOR('',#35407,1000.);
#9284=VECTOR('',#35412,1000.);
#9285=VECTOR('',#35413,1000.);
#9286=VECTOR('',#35416,1000.);
#9287=VECTOR('',#35421,1000.);
#9288=VECTOR('',#35424,1000.);
#9289=VECTOR('',#35427,1000.);
#10459=CIRCLE('',#28268,26.);
#10460=CIRCLE('',#28269,9.5);
#10461=CIRCLE('',#28271,27.5);
#10462=CIRCLE('',#28273,13.);
#10463=CIRCLE('',#28274,27.5);
#10464=CIRCLE('',#28275,13.);
#10465=CIRCLE('',#28276,17.5);
#10466=CIRCLE('',#28278,13.);
#10467=CIRCLE('',#28279,27.5);
#10468=CIRCLE('',#28280,13.);
#10469=CIRCLE('',#28281,17.5);
#10470=CIRCLE('',#28283,17.5);
#10471=CIRCLE('',#28285,17.5);
#10472=CIRCLE('',#28287,13.);
#10473=CIRCLE('',#28289,13.);
#10474=CIRCLE('',#28291,13.);
#10475=CIRCLE('',#28293,13.);
#10476=CIRCLE('',#28295,27.5);
#10477=CIRCLE('',#28296,27.5);
#10478=CIRCLE('',#28297,27.5);
#10479=CIRCLE('',#28299,9.5);
#10480=CIRCLE('',#28302,2.5);
#10481=CIRCLE('',#28304,5.5);
#10482=CIRCLE('',#28305,3.3);
#10483=CIRCLE('',#28307,3.3);
#10484=CIRCLE('',#28309,2.5);
#10485=CIRCLE('',#28311,2.5);
#10486=CIRCLE('',#28316,5.5);
#10487=CIRCLE('',#28318,2.5);
#10488=CIRCLE('',#28321,2.5);
#10489=CIRCLE('',#28322,2.5);
#10490=CIRCLE('',#28324,3.3);
#10491=CIRCLE('',#28326,3.3);
#10492=CIRCLE('',#28330,9.5);
#10493=CIRCLE('',#28331,9.5);
#10494=CIRCLE('',#28332,26.);
#10495=CIRCLE('',#28334,27.5);
#10496=CIRCLE('',#28336,27.5);
#10497=CIRCLE('',#28337,13.);
#10498=CIRCLE('',#28338,17.5);
#10499=CIRCLE('',#28339,13.);
#10500=CIRCLE('',#28340,27.5);
#10501=CIRCLE('',#28341,13.);
#10502=CIRCLE('',#28342,17.5);
#10503=CIRCLE('',#28343,13.);
#10504=CIRCLE('',#28344,27.5);
#10505=CIRCLE('',#28345,9.5);
#10506=CIRCLE('',#28346,9.5);
#10507=CIRCLE('',#28350,27.5);
#10508=CIRCLE('',#28352,2.1);
#10509=CIRCLE('',#28357,13.);
#10510=CIRCLE('',#28359,13.);
#10511=CIRCLE('',#28361,13.);
#10512=CIRCLE('',#28363,17.5);
#10513=CIRCLE('',#28365,17.5);
#10514=CIRCLE('',#28367,13.);
#10515=CIRCLE('',#28369,27.5);
#10516=CIRCLE('',#28371,27.5);
#10517=CIRCLE('',#28373,30.7157076295626);
#10518=CIRCLE('',#28374,30.7139923779046);
#10519=CIRCLE('',#28375,27.5);
#10520=CIRCLE('',#28376,27.5);
#10521=CIRCLE('',#28377,27.5);
#10522=CIRCLE('',#28378,27.5);
#10523=CIRCLE('',#28379,27.5);
#10524=CIRCLE('',#28380,27.5);
#10525=CIRCLE('',#28386,37.5686105495472);
#10526=CIRCLE('',#28387,27.5);
#10527=CIRCLE('',#28388,27.5);
#10528=CIRCLE('',#28389,27.5);
#10529=CIRCLE('',#28390,39.9577086923309);
#10530=CIRCLE('',#28397,27.);
#10531=CIRCLE('',#28398,27.);
#10532=CIRCLE('',#28399,27.);
#10533=CIRCLE('',#28400,27.);
#10534=CIRCLE('',#28416,39.2292319120603);
#10535=CIRCLE('',#28418,27.);
#10536=CIRCLE('',#28421,27.);
#10537=CIRCLE('',#28424,27.);
#10538=CIRCLE('',#28451,30.15506861437);
#10539=CIRCLE('',#28454,30.1568155811663);
#10540=CIRCLE('',#28458,27.);
#10541=CIRCLE('',#28461,27.);
#10542=CIRCLE('',#28464,27.);
#12639=VERTEX_POINT('',#65195);
#12640=VERTEX_POINT('',#65196);
#12641=VERTEX_POINT('',#65198);
#12642=VERTEX_POINT('',#65200);
#12643=VERTEX_POINT('',#65204);
#12644=VERTEX_POINT('',#65205);
#12645=VERTEX_POINT('',#65210);
#12646=VERTEX_POINT('',#65211);
#12647=VERTEX_POINT('',#65213);
#12648=VERTEX_POINT('',#65215);
#12649=VERTEX_POINT('',#65219);
#12650=VERTEX_POINT('',#65220);
#12651=VERTEX_POINT('',#65222);
#12652=VERTEX_POINT('',#65224);
#12653=VERTEX_POINT('',#65228);
#12654=VERTEX_POINT('',#65229);
#12655=VERTEX_POINT('',#65234);
#12656=VERTEX_POINT('',#65236);
#12657=VERTEX_POINT('',#65240);
#12658=VERTEX_POINT('',#65244);
#12659=VERTEX_POINT('',#65248);
#12660=VERTEX_POINT('',#65252);
#12661=VERTEX_POINT('',#65257);
#12662=VERTEX_POINT('',#65260);
#12663=VERTEX_POINT('',#65263);
#12664=VERTEX_POINT('',#65264);
#12665=VERTEX_POINT('',#65308);
#12666=VERTEX_POINT('',#65309);
#12667=VERTEX_POINT('',#65342);
#12668=VERTEX_POINT('',#65344);
#12669=VERTEX_POINT('',#65351);
#12670=VERTEX_POINT('',#65356);
#12671=VERTEX_POINT('',#65359);
#12672=VERTEX_POINT('',#65363);
#12673=VERTEX_POINT('',#65366);
#12674=VERTEX_POINT('',#65373);
#12675=VERTEX_POINT('',#65374);
#12676=VERTEX_POINT('',#65407);
#12677=VERTEX_POINT('',#65408);
#12678=VERTEX_POINT('',#65410);
#12679=VERTEX_POINT('',#65412);
#12680=VERTEX_POINT('',#65414);
#12681=VERTEX_POINT('',#65417);
#12682=VERTEX_POINT('',#65420);
#12683=VERTEX_POINT('',#65421);
#12684=VERTEX_POINT('',#65464);
#12685=VERTEX_POINT('',#65466);
#12686=VERTEX_POINT('',#65470);
#12687=VERTEX_POINT('',#65473);
#12688=VERTEX_POINT('',#65479);
#12689=VERTEX_POINT('',#65480);
#12690=VERTEX_POINT('',#65482);
#12691=VERTEX_POINT('',#65484);
#12692=VERTEX_POINT('',#65486);
#12693=VERTEX_POINT('',#65490);
#12694=VERTEX_POINT('',#65492);
#12695=VERTEX_POINT('',#65494);
#12696=VERTEX_POINT('',#65496);
#12697=VERTEX_POINT('',#65503);
#12698=VERTEX_POINT('',#65505);
#12699=VERTEX_POINT('',#65507);
#12700=VERTEX_POINT('',#65509);
#12701=VERTEX_POINT('',#65511);
#12702=VERTEX_POINT('',#65513);
#12703=VERTEX_POINT('',#65515);
#12704=VERTEX_POINT('',#65517);
#12705=VERTEX_POINT('',#65520);
#12706=VERTEX_POINT('',#65522);
#12707=VERTEX_POINT('',#65524);
#12708=VERTEX_POINT('',#65526);
#12709=VERTEX_POINT('',#65534);
#12710=VERTEX_POINT('',#65535);
#12711=VERTEX_POINT('',#65537);
#12712=VERTEX_POINT('',#65556);
#12713=VERTEX_POINT('',#65560);
#12714=VERTEX_POINT('',#65562);
#12715=VERTEX_POINT('',#65564);
#12716=VERTEX_POINT('',#65583);
#12717=VERTEX_POINT('',#65661);
#12718=VERTEX_POINT('',#65662);
#12719=VERTEX_POINT('',#65667);
#12720=VERTEX_POINT('',#65668);
#12721=VERTEX_POINT('',#65673);
#12722=VERTEX_POINT('',#65675);
#12723=VERTEX_POINT('',#65679);
#12724=VERTEX_POINT('',#65685);
#12725=VERTEX_POINT('',#65693);
#12726=VERTEX_POINT('',#65694);
#12727=VERTEX_POINT('',#65711);
#12728=VERTEX_POINT('',#65713);
#12729=VERTEX_POINT('',#65715);
#12730=VERTEX_POINT('',#65717);
#12731=VERTEX_POINT('',#65719);
#12732=VERTEX_POINT('',#65721);
#12733=VERTEX_POINT('',#65723);
#12734=VERTEX_POINT('',#65726);
#12735=VERTEX_POINT('',#65727);
#12736=VERTEX_POINT('',#65729);
#12737=VERTEX_POINT('',#65731);
#12738=VERTEX_POINT('',#65733);
#12739=VERTEX_POINT('',#65735);
#12740=VERTEX_POINT('',#65737);
#12741=VERTEX_POINT('',#65739);
#12742=VERTEX_POINT('',#65742);
#12743=VERTEX_POINT('',#65743);
#12744=VERTEX_POINT('',#65745);
#12745=VERTEX_POINT('',#65747);
#12746=VERTEX_POINT('',#65749);
#12747=VERTEX_POINT('',#65751);
#12748=VERTEX_POINT('',#65754);
#12749=VERTEX_POINT('',#65755);
#12750=VERTEX_POINT('',#65757);
#12751=VERTEX_POINT('',#65759);
#12752=VERTEX_POINT('',#65761);
#12753=VERTEX_POINT('',#65763);
#12754=VERTEX_POINT('',#65765);
#12755=VERTEX_POINT('',#65767);
#12756=VERTEX_POINT('',#65769);
#12757=VERTEX_POINT('',#65771);
#12758=VERTEX_POINT('',#65773);
#12759=VERTEX_POINT('',#65776);
#12760=VERTEX_POINT('',#65777);
#12761=VERTEX_POINT('',#65779);
#12762=VERTEX_POINT('',#65781);
#12763=VERTEX_POINT('',#65783);
#12764=VERTEX_POINT('',#65785);
#12765=VERTEX_POINT('',#65789);
#12766=VERTEX_POINT('',#65790);
#12767=VERTEX_POINT('',#65792);
#12768=VERTEX_POINT('',#65794);
#12769=VERTEX_POINT('',#65796);
#12770=VERTEX_POINT('',#65798);
#12771=VERTEX_POINT('',#65800);
#12772=VERTEX_POINT('',#65802);
#12773=VERTEX_POINT('',#65822);
#12774=VERTEX_POINT('',#65824);
#12775=VERTEX_POINT('',#65828);
#12776=VERTEX_POINT('',#65832);
#12777=VERTEX_POINT('',#65836);
#12778=VERTEX_POINT('',#65838);
#12779=VERTEX_POINT('',#65842);
#12780=VERTEX_POINT('',#65846);
#12781=VERTEX_POINT('',#65850);
#12782=VERTEX_POINT('',#65854);
#12783=VERTEX_POINT('',#65858);
#12784=VERTEX_POINT('',#65867);
#12785=VERTEX_POINT('',#65868);
#12786=VERTEX_POINT('',#65870);
#12787=VERTEX_POINT('',#65872);
#12788=VERTEX_POINT('',#65874);
#12789=VERTEX_POINT('',#65876);
#12790=VERTEX_POINT('',#65892);
#12791=VERTEX_POINT('',#65894);
#12792=VERTEX_POINT('',#65898);
#12793=VERTEX_POINT('',#65902);
#12794=VERTEX_POINT('',#65906);
#12795=VERTEX_POINT('',#65910);
#12796=VERTEX_POINT('',#65917);
#12797=VERTEX_POINT('',#65919);
#12798=VERTEX_POINT('',#65923);
#12799=VERTEX_POINT('',#65927);
#12800=VERTEX_POINT('',#65931);
#12801=VERTEX_POINT('',#65950);
#12802=VERTEX_POINT('',#65954);
#12803=VERTEX_POINT('',#65956);
#12804=VERTEX_POINT('',#65960);
#12805=VERTEX_POINT('',#65964);
#12806=VERTEX_POINT('',#65968);
#12807=VERTEX_POINT('',#65972);
#12808=VERTEX_POINT('',#65978);
#16075=EDGE_CURVE('',#12639,#12640,#7166,.T.);
#16076=EDGE_CURVE('',#12640,#12641,#10459,.T.);
#16077=EDGE_CURVE('',#12641,#12642,#7167,.T.);
#16078=EDGE_CURVE('',#12642,#12639,#10460,.T.);
#16079=EDGE_CURVE('',#12643,#12644,#10461,.T.);
#16080=EDGE_CURVE('',#12644,#12641,#7168,.T.);
#16081=EDGE_CURVE('',#12640,#12643,#7169,.T.);
#16082=EDGE_CURVE('',#12645,#12646,#10462,.T.);
#16083=EDGE_CURVE('',#12647,#12646,#10463,.T.);
#16084=EDGE_CURVE('',#12647,#12648,#10464,.T.);
#16085=EDGE_CURVE('',#12648,#12645,#10465,.T.);
#16086=EDGE_CURVE('',#12649,#12650,#10466,.T.);
#16087=EDGE_CURVE('',#12651,#12650,#10467,.T.);
#16088=EDGE_CURVE('',#12651,#12652,#10468,.T.);
#16089=EDGE_CURVE('',#12652,#12649,#10469,.T.);
#16090=EDGE_CURVE('',#12653,#12654,#10470,.T.);
#16091=EDGE_CURVE('',#12654,#12649,#7170,.T.);
#16092=EDGE_CURVE('',#12652,#12653,#7171,.T.);
#16093=EDGE_CURVE('',#12655,#12645,#7172,.T.);
#16094=EDGE_CURVE('',#12648,#12656,#7173,.T.);
#16095=EDGE_CURVE('',#12656,#12655,#10471,.T.);
#16096=EDGE_CURVE('',#12657,#12651,#7174,.T.);
#16097=EDGE_CURVE('',#12657,#12653,#10472,.T.);
#16098=EDGE_CURVE('',#12658,#12647,#7175,.T.);
#16099=EDGE_CURVE('',#12658,#12656,#10473,.T.);
#16100=EDGE_CURVE('',#12654,#12659,#10474,.T.);
#16101=EDGE_CURVE('',#12650,#12659,#7176,.T.);
#16102=EDGE_CURVE('',#12655,#12660,#10475,.T.);
#16103=EDGE_CURVE('',#12646,#12660,#7177,.T.);
#16104=EDGE_CURVE('',#12659,#12658,#10476,.T.);
#16105=EDGE_CURVE('',#12660,#12661,#10477,.T.);
#16106=EDGE_CURVE('',#12661,#12644,#7178,.T.);
#16107=EDGE_CURVE('',#12643,#12662,#7179,.T.);
#16108=EDGE_CURVE('',#12662,#12657,#10478,.T.);
#16109=EDGE_CURVE('',#12663,#12664,#389,.T.);
#16110=EDGE_CURVE('',#12664,#12663,#390,.T.);
#16111=EDGE_CURVE('',#12665,#12666,#7180,.T.);
#16112=EDGE_CURVE('',#12666,#12665,#391,.T.);
#16113=EDGE_CURVE('',#12642,#12667,#7181,.T.);
#16114=EDGE_CURVE('',#12668,#12667,#10479,.T.);
#16115=EDGE_CURVE('',#12668,#12639,#7182,.T.);
#16116=EDGE_CURVE('',#12662,#12668,#7183,.T.);
#16117=EDGE_CURVE('',#12667,#12661,#7184,.T.);
#16118=EDGE_CURVE('',#12664,#12669,#7185,.T.);
#16119=EDGE_CURVE('',#12669,#12669,#10480,.T.);
#16120=EDGE_CURVE('',#12665,#12666,#10481,.T.);
#16121=EDGE_CURVE('',#12670,#12670,#10482,.T.);
#16122=EDGE_CURVE('',#12671,#12671,#10483,.T.);
#16123=EDGE_CURVE('',#12671,#12670,#7186,.T.);
#16124=EDGE_CURVE('',#12672,#12672,#10484,.T.);
#16125=EDGE_CURVE('',#12673,#12673,#10485,.T.);
#16126=EDGE_CURVE('',#12673,#12672,#7187,.T.);
#16127=EDGE_CURVE('',#12674,#12675,#10486,.T.);
#16128=EDGE_CURVE('',#12675,#12674,#392,.F.);
#16129=EDGE_CURVE('',#12676,#12677,#7188,.T.);
#16130=EDGE_CURVE('',#12678,#12676,#7189,.T.);
#16131=EDGE_CURVE('',#12679,#12678,#7190,.T.);
#16132=EDGE_CURVE('',#12680,#12679,#7191,.T.);
#16133=EDGE_CURVE('',#12677,#12680,#7192,.T.);
#16134=EDGE_CURVE('',#12681,#12681,#10487,.T.);
#16135=EDGE_CURVE('',#12682,#12683,#393,.F.);
#16136=EDGE_CURVE('',#12683,#12682,#394,.F.);
#16137=EDGE_CURVE('',#12683,#12681,#7193,.T.);
#16138=EDGE_CURVE('',#12684,#12684,#10488,.T.);
#16139=EDGE_CURVE('',#12684,#12685,#7194,.T.);
#16140=EDGE_CURVE('',#12685,#12685,#10489,.T.);
#16141=EDGE_CURVE('',#12686,#12686,#10490,.T.);
#16142=EDGE_CURVE('',#12686,#12687,#7195,.T.);
#16143=EDGE_CURVE('',#12687,#12687,#10491,.T.);
#16144=EDGE_CURVE('',#12674,#12675,#7196,.T.);
#16145=EDGE_CURVE('',#12688,#12689,#7197,.T.);
#16146=EDGE_CURVE('',#12690,#12688,#7198,.T.);
#16147=EDGE_CURVE('',#12691,#12690,#7199,.T.);
#16148=EDGE_CURVE('',#12692,#12691,#7200,.T.);
#16149=EDGE_CURVE('',#12689,#12692,#7201,.T.);
#16150=EDGE_CURVE('',#12692,#12693,#10492,.T.);
#16151=EDGE_CURVE('',#12693,#12694,#7202,.T.);
#16152=EDGE_CURVE('',#12694,#12695,#7203,.T.);
#16153=EDGE_CURVE('',#12695,#12696,#7204,.T.);
#16154=EDGE_CURVE('',#12696,#12678,#10493,.T.);
#16155=EDGE_CURVE('',#12676,#12689,#10494,.T.);
#16156=EDGE_CURVE('',#12677,#12688,#10495,.T.);
#16157=EDGE_CURVE('',#12697,#12690,#10496,.T.);
#16158=EDGE_CURVE('',#12698,#12697,#10497,.T.);
#16159=EDGE_CURVE('',#12699,#12698,#10498,.T.);
#16160=EDGE_CURVE('',#12700,#12699,#10499,.T.);
#16161=EDGE_CURVE('',#12701,#12700,#10500,.T.);
#16162=EDGE_CURVE('',#12702,#12701,#10501,.T.);
#16163=EDGE_CURVE('',#12703,#12702,#10502,.T.);
#16164=EDGE_CURVE('',#12704,#12703,#10503,.T.);
#16165=EDGE_CURVE('',#12680,#12704,#10504,.T.);
#16166=EDGE_CURVE('',#12679,#12705,#10505,.T.);
#16167=EDGE_CURVE('',#12705,#12706,#7205,.T.);
#16168=EDGE_CURVE('',#12706,#12707,#7206,.T.);
#16169=EDGE_CURVE('',#12707,#12708,#7207,.T.);
#16170=EDGE_CURVE('',#12708,#12691,#10506,.T.);
#16171=EDGE_CURVE('',#12705,#12696,#7208,.T.);
#16172=EDGE_CURVE('',#12693,#12708,#7209,.T.);
#16173=EDGE_CURVE('',#12709,#12710,#7210,.T.);
#16174=EDGE_CURVE('',#12710,#12711,#395,.T.);
#16175=EDGE_CURVE('',#12711,#12712,#7211,.T.);
#16176=EDGE_CURVE('',#12712,#12709,#10507,.T.);
#16177=EDGE_CURVE('',#12713,#12713,#10508,.T.);
#16178=EDGE_CURVE('',#12713,#12714,#7212,.T.);
#16179=EDGE_CURVE('',#12715,#12714,#396,.T.);
#16180=EDGE_CURVE('',#12716,#12715,#397,.T.);
#16181=EDGE_CURVE('',#12714,#12716,#398,.T.);
#16182=EDGE_CURVE('',#12707,#12694,#7213,.T.);
#16183=EDGE_CURVE('',#12695,#12706,#7214,.T.);
#16184=EDGE_CURVE('',#12717,#12718,#10509,.T.);
#16185=EDGE_CURVE('',#12704,#12717,#7215,.T.);
#16186=EDGE_CURVE('',#12718,#12703,#7216,.T.);
#16187=EDGE_CURVE('',#12719,#12720,#10510,.T.);
#16188=EDGE_CURVE('',#12700,#12719,#7217,.T.);
#16189=EDGE_CURVE('',#12720,#12699,#7218,.T.);
#16190=EDGE_CURVE('',#12721,#12697,#7219,.T.);
#16191=EDGE_CURVE('',#12722,#12721,#10511,.T.);
#16192=EDGE_CURVE('',#12698,#12722,#7220,.T.);
#16193=EDGE_CURVE('',#12718,#12723,#10512,.T.);
#16194=EDGE_CURVE('',#12702,#12723,#7221,.T.);
#16195=EDGE_CURVE('',#12720,#12722,#10513,.T.);
#16196=EDGE_CURVE('',#12724,#12701,#7222,.T.);
#16197=EDGE_CURVE('',#12723,#12724,#10514,.T.);
#16198=EDGE_CURVE('',#12719,#12721,#10515,.T.);
#16199=EDGE_CURVE('',#12717,#12724,#10516,.T.);
#16200=EDGE_CURVE('',#12725,#12726,#399,.F.);
#16201=EDGE_CURVE('',#12726,#12727,#10517,.T.);
#16202=EDGE_CURVE('',#12727,#12728,#7223,.T.);
#16203=EDGE_CURVE('',#12728,#12729,#10518,.T.);
#16204=EDGE_CURVE('',#12729,#12730,#7224,.T.);
#16205=EDGE_CURVE('',#12730,#12731,#10519,.T.);
#16206=EDGE_CURVE('',#12731,#12732,#7225,.T.);
#16207=EDGE_CURVE('',#12732,#12733,#10520,.T.);
#16208=EDGE_CURVE('',#12733,#12725,#7226,.T.);
#16209=EDGE_CURVE('',#12734,#12735,#10521,.T.);
#16210=EDGE_CURVE('',#12735,#12736,#7227,.T.);
#16211=EDGE_CURVE('',#12736,#12737,#10522,.T.);
#16212=EDGE_CURVE('',#12737,#12738,#7228,.T.);
#16213=EDGE_CURVE('',#12738,#12739,#10523,.T.);
#16214=EDGE_CURVE('',#12739,#12740,#7229,.T.);
#16215=EDGE_CURVE('',#12740,#12741,#10524,.T.);
#16216=EDGE_CURVE('',#12741,#12734,#7230,.T.);
#16217=EDGE_CURVE('',#12742,#12743,#7231,.T.);
#16218=EDGE_CURVE('',#12743,#12744,#679,.T.);
#16219=EDGE_CURVE('',#12744,#12745,#680,.T.);
#16220=EDGE_CURVE('',#12745,#12746,#7232,.T.);
#16221=EDGE_CURVE('',#12746,#12747,#681,.T.);
#16222=EDGE_CURVE('',#12747,#12742,#682,.T.);
#16223=EDGE_CURVE('',#12748,#12749,#683,.F.);
#16224=EDGE_CURVE('',#12749,#12750,#7233,.T.);
#16225=EDGE_CURVE('',#12750,#12751,#10525,.T.);
#16226=EDGE_CURVE('',#12751,#12752,#10526,.T.);
#16227=EDGE_CURVE('',#12752,#12753,#7234,.T.);
#16228=EDGE_CURVE('',#12753,#12754,#10527,.T.);
#16229=EDGE_CURVE('',#12754,#12755,#7235,.T.);
#16230=EDGE_CURVE('',#12755,#12756,#10528,.T.);
#16231=EDGE_CURVE('',#12756,#12757,#10529,.T.);
#16232=EDGE_CURVE('',#12757,#12758,#7236,.T.);
#16233=EDGE_CURVE('',#12758,#12748,#684,.T.);
#16234=EDGE_CURVE('',#12759,#12760,#685,.T.);
#16235=EDGE_CURVE('',#12760,#12761,#7237,.T.);
#16236=EDGE_CURVE('',#12761,#12762,#686,.T.);
#16237=EDGE_CURVE('',#12762,#12763,#687,.T.);
#16238=EDGE_CURVE('',#12763,#12764,#7238,.T.);
#16239=EDGE_CURVE('',#12764,#12759,#688,.T.);
#16240=EDGE_CURVE('',#12765,#12766,#10530,.T.);
#16241=EDGE_CURVE('',#12766,#12767,#7239,.T.);
#16242=EDGE_CURVE('',#12767,#12768,#10531,.T.);
#16243=EDGE_CURVE('',#12768,#12769,#7240,.T.);
#16244=EDGE_CURVE('',#12769,#12770,#10532,.T.);
#16245=EDGE_CURVE('',#12770,#12771,#7241,.T.);
#16246=EDGE_CURVE('',#12771,#12772,#10533,.T.);
#16247=EDGE_CURVE('',#12772,#12765,#7242,.T.);
#16248=EDGE_CURVE('',#12772,#12736,#7243,.T.);
#16249=EDGE_CURVE('',#12771,#12737,#7244,.T.);
#16250=EDGE_CURVE('',#12765,#12735,#7245,.T.);
#16251=EDGE_CURVE('',#12770,#12738,#7246,.T.);
#16252=EDGE_CURVE('',#12769,#12739,#7247,.T.);
#16253=EDGE_CURVE('',#12768,#12740,#7248,.T.);
#16254=EDGE_CURVE('',#12767,#12741,#7249,.T.);
#16255=EDGE_CURVE('',#12766,#12734,#7250,.T.);
#16256=EDGE_CURVE('',#12773,#12750,#7251,.T.);
#16257=EDGE_CURVE('',#12774,#12773,#689,.T.);
#16258=EDGE_CURVE('',#12774,#12751,#7252,.T.);
#16259=EDGE_CURVE('',#12775,#12749,#7253,.T.);
#16260=EDGE_CURVE('',#12773,#12775,#7254,.T.);
#16261=EDGE_CURVE('',#12776,#12748,#7255,.T.);
#16262=EDGE_CURVE('',#12775,#12776,#690,.F.);
#16263=EDGE_CURVE('',#12777,#12757,#7256,.T.);
#16264=EDGE_CURVE('',#12778,#12777,#7257,.T.);
#16265=EDGE_CURVE('',#12778,#12758,#7258,.T.);
#16266=EDGE_CURVE('',#12779,#12756,#7259,.T.);
#16267=EDGE_CURVE('',#12777,#12779,#10534,.T.);
#16268=EDGE_CURVE('',#12780,#12755,#7260,.T.);
#16269=EDGE_CURVE('',#12779,#12780,#10535,.T.);
#16270=EDGE_CURVE('',#12781,#12754,#7261,.T.);
#16271=EDGE_CURVE('',#12780,#12781,#7262,.T.);
#16272=EDGE_CURVE('',#12782,#12753,#7263,.T.);
#16273=EDGE_CURVE('',#12781,#12782,#10536,.T.);
#16274=EDGE_CURVE('',#12783,#12752,#7264,.T.);
#16275=EDGE_CURVE('',#12782,#12783,#7265,.T.);
#16276=EDGE_CURVE('',#12783,#12774,#10537,.T.);
#16277=EDGE_CURVE('',#12776,#12778,#691,.T.);
#16278=EDGE_CURVE('',#12784,#12785,#692,.T.);
#16279=EDGE_CURVE('',#12785,#12786,#7266,.T.);
#16280=EDGE_CURVE('',#12786,#12787,#693,.T.);
#16281=EDGE_CURVE('',#12787,#12788,#694,.T.);
#16282=EDGE_CURVE('',#12788,#12789,#7267,.T.);
#16283=EDGE_CURVE('',#12789,#12784,#695,.T.);
#16284=EDGE_CURVE('',#12787,#12744,#7268,.T.);
#16285=EDGE_CURVE('',#12786,#12745,#7269,.T.);
#16286=EDGE_CURVE('',#12788,#12743,#7270,.T.);
#16287=EDGE_CURVE('',#12785,#12746,#7271,.T.);
#16288=EDGE_CURVE('',#12784,#12747,#7272,.T.);
#16289=EDGE_CURVE('',#12789,#12742,#7273,.T.);
#16290=EDGE_CURVE('',#12790,#12763,#7274,.T.);
#16291=EDGE_CURVE('',#12791,#12790,#7275,.T.);
#16292=EDGE_CURVE('',#12791,#12764,#7276,.T.);
#16293=EDGE_CURVE('',#12792,#12762,#7277,.T.);
#16294=EDGE_CURVE('',#12790,#12792,#696,.T.);
#16295=EDGE_CURVE('',#12793,#12761,#7278,.T.);
#16296=EDGE_CURVE('',#12792,#12793,#697,.T.);
#16297=EDGE_CURVE('',#12794,#12760,#7279,.T.);
#16298=EDGE_CURVE('',#12793,#12794,#7280,.T.);
#16299=EDGE_CURVE('',#12795,#12791,#698,.T.);
#16300=EDGE_CURVE('',#12795,#12759,#7281,.T.);
#16301=EDGE_CURVE('',#12794,#12795,#699,.T.);
#16302=EDGE_CURVE('',#12796,#12728,#7282,.T.);
#16303=EDGE_CURVE('',#12797,#12796,#10538,.T.);
#16304=EDGE_CURVE('',#12797,#12729,#7283,.T.);
#16305=EDGE_CURVE('',#12798,#12727,#7284,.T.);
#16306=EDGE_CURVE('',#12796,#12798,#7285,.T.);
#16307=EDGE_CURVE('',#12799,#12726,#7286,.T.);
#16308=EDGE_CURVE('',#12798,#12799,#10539,.T.);
#16309=EDGE_CURVE('',#12800,#12725,#7287,.T.);
#16310=EDGE_CURVE('',#12799,#12800,#400,.F.);
#16311=EDGE_CURVE('',#12801,#12733,#7288,.T.);
#16312=EDGE_CURVE('',#12800,#12801,#7289,.T.);
#16313=EDGE_CURVE('',#12802,#12712,#7290,.T.);
#16314=EDGE_CURVE('',#12803,#12802,#10540,.T.);
#16315=EDGE_CURVE('',#12803,#12709,#7291,.T.);
#16316=EDGE_CURVE('',#12804,#12711,#7292,.T.);
#16317=EDGE_CURVE('',#12802,#12804,#7293,.T.);
#16318=EDGE_CURVE('',#12805,#12732,#7294,.T.);
#16319=EDGE_CURVE('',#12801,#12805,#10541,.T.);
#16320=EDGE_CURVE('',#12806,#12731,#7295,.T.);
#16321=EDGE_CURVE('',#12805,#12806,#7296,.T.);
#16322=EDGE_CURVE('',#12807,#12730,#7297,.T.);
#16323=EDGE_CURVE('',#12806,#12807,#10542,.T.);
#16324=EDGE_CURVE('',#12807,#12797,#7298,.T.);
#16325=EDGE_CURVE('',#12808,#12710,#7299,.T.);
#16326=EDGE_CURVE('',#12804,#12808,#401,.T.);
#16327=EDGE_CURVE('',#12808,#12803,#7300,.T.);
#22764=ORIENTED_EDGE('',*,*,#16075,.T.);
#22765=ORIENTED_EDGE('',*,*,#16076,.T.);
#22766=ORIENTED_EDGE('',*,*,#16077,.T.);
#22767=ORIENTED_EDGE('',*,*,#16078,.T.);
#22768=ORIENTED_EDGE('',*,*,#16079,.T.);
#22769=ORIENTED_EDGE('',*,*,#16080,.T.);
#22770=ORIENTED_EDGE('',*,*,#16076,.F.);
#22771=ORIENTED_EDGE('',*,*,#16081,.T.);
#22772=ORIENTED_EDGE('',*,*,#16082,.T.);
#22773=ORIENTED_EDGE('',*,*,#16083,.F.);
#22774=ORIENTED_EDGE('',*,*,#16084,.T.);
#22775=ORIENTED_EDGE('',*,*,#16085,.T.);
#22776=ORIENTED_EDGE('',*,*,#16086,.T.);
#22777=ORIENTED_EDGE('',*,*,#16087,.F.);
#22778=ORIENTED_EDGE('',*,*,#16088,.T.);
#22779=ORIENTED_EDGE('',*,*,#16089,.T.);
#22780=ORIENTED_EDGE('',*,*,#16090,.T.);
#22781=ORIENTED_EDGE('',*,*,#16091,.T.);
#22782=ORIENTED_EDGE('',*,*,#16089,.F.);
#22783=ORIENTED_EDGE('',*,*,#16092,.T.);
#22784=ORIENTED_EDGE('',*,*,#16093,.T.);
#22785=ORIENTED_EDGE('',*,*,#16085,.F.);
#22786=ORIENTED_EDGE('',*,*,#16094,.T.);
#22787=ORIENTED_EDGE('',*,*,#16095,.T.);
#22788=ORIENTED_EDGE('',*,*,#16088,.F.);
#22789=ORIENTED_EDGE('',*,*,#16096,.F.);
#22790=ORIENTED_EDGE('',*,*,#16097,.T.);
#22791=ORIENTED_EDGE('',*,*,#16092,.F.);
#22792=ORIENTED_EDGE('',*,*,#16084,.F.);
#22793=ORIENTED_EDGE('',*,*,#16098,.F.);
#22794=ORIENTED_EDGE('',*,*,#16099,.T.);
#22795=ORIENTED_EDGE('',*,*,#16094,.F.);
#22796=ORIENTED_EDGE('',*,*,#16100,.T.);
#22797=ORIENTED_EDGE('',*,*,#16101,.F.);
#22798=ORIENTED_EDGE('',*,*,#16086,.F.);
#22799=ORIENTED_EDGE('',*,*,#16091,.F.);
#22800=ORIENTED_EDGE('',*,*,#16102,.T.);
#22801=ORIENTED_EDGE('',*,*,#16103,.F.);
#22802=ORIENTED_EDGE('',*,*,#16082,.F.);
#22803=ORIENTED_EDGE('',*,*,#16093,.F.);
#22804=ORIENTED_EDGE('',*,*,#16087,.T.);
#22805=ORIENTED_EDGE('',*,*,#16101,.T.);
#22806=ORIENTED_EDGE('',*,*,#16104,.T.);
#22807=ORIENTED_EDGE('',*,*,#16098,.T.);
#22808=ORIENTED_EDGE('',*,*,#16083,.T.);
#22809=ORIENTED_EDGE('',*,*,#16103,.T.);
#22810=ORIENTED_EDGE('',*,*,#16105,.T.);
#22811=ORIENTED_EDGE('',*,*,#16106,.T.);
#22812=ORIENTED_EDGE('',*,*,#16079,.F.);
#22813=ORIENTED_EDGE('',*,*,#16107,.T.);
#22814=ORIENTED_EDGE('',*,*,#16108,.T.);
#22815=ORIENTED_EDGE('',*,*,#16096,.T.);
#22816=ORIENTED_EDGE('',*,*,#16109,.T.);
#22817=ORIENTED_EDGE('',*,*,#16110,.T.);
#22818=ORIENTED_EDGE('',*,*,#16111,.T.);
#22819=ORIENTED_EDGE('',*,*,#16112,.T.);
#22820=ORIENTED_EDGE('',*,*,#16078,.F.);
#22821=ORIENTED_EDGE('',*,*,#16113,.T.);
#22822=ORIENTED_EDGE('',*,*,#16114,.F.);
#22823=ORIENTED_EDGE('',*,*,#16115,.T.);
#22824=ORIENTED_EDGE('',*,*,#16116,.T.);
#22825=ORIENTED_EDGE('',*,*,#16114,.T.);
#22826=ORIENTED_EDGE('',*,*,#16117,.T.);
#22827=ORIENTED_EDGE('',*,*,#16105,.F.);
#22828=ORIENTED_EDGE('',*,*,#16102,.F.);
#22829=ORIENTED_EDGE('',*,*,#16095,.F.);
#22830=ORIENTED_EDGE('',*,*,#16099,.F.);
#22831=ORIENTED_EDGE('',*,*,#16104,.F.);
#22832=ORIENTED_EDGE('',*,*,#16100,.F.);
#22833=ORIENTED_EDGE('',*,*,#16090,.F.);
#22834=ORIENTED_EDGE('',*,*,#16097,.F.);
#22835=ORIENTED_EDGE('',*,*,#16108,.F.);
#22836=ORIENTED_EDGE('',*,*,#16109,.F.);
#22837=ORIENTED_EDGE('',*,*,#16110,.F.);
#22838=ORIENTED_EDGE('',*,*,#16118,.T.);
#22839=ORIENTED_EDGE('',*,*,#16119,.T.);
#22840=ORIENTED_EDGE('',*,*,#16118,.F.);
#22841=ORIENTED_EDGE('',*,*,#16111,.F.);
#22842=ORIENTED_EDGE('',*,*,#16120,.T.);
#22843=ORIENTED_EDGE('',*,*,#16121,.F.);
#22844=ORIENTED_EDGE('',*,*,#16122,.F.);
#22845=ORIENTED_EDGE('',*,*,#16123,.T.);
#22846=ORIENTED_EDGE('',*,*,#16121,.T.);
#22847=ORIENTED_EDGE('',*,*,#16123,.F.);
#22848=ORIENTED_EDGE('',*,*,#16122,.T.);
#22849=ORIENTED_EDGE('',*,*,#16124,.F.);
#22850=ORIENTED_EDGE('',*,*,#16125,.T.);
#22851=ORIENTED_EDGE('',*,*,#16126,.T.);
#22852=ORIENTED_EDGE('',*,*,#16124,.T.);
#22853=ORIENTED_EDGE('',*,*,#16126,.F.);
#22854=ORIENTED_EDGE('',*,*,#16081,.F.);
#22855=ORIENTED_EDGE('',*,*,#16075,.F.);
#22856=ORIENTED_EDGE('',*,*,#16115,.F.);
#22857=ORIENTED_EDGE('',*,*,#16116,.F.);
#22858=ORIENTED_EDGE('',*,*,#16107,.F.);
#22859=ORIENTED_EDGE('',*,*,#16119,.F.);
#22860=ORIENTED_EDGE('',*,*,#16080,.F.);
#22861=ORIENTED_EDGE('',*,*,#16106,.F.);
#22862=ORIENTED_EDGE('',*,*,#16117,.F.);
#22863=ORIENTED_EDGE('',*,*,#16113,.F.);
#22864=ORIENTED_EDGE('',*,*,#16077,.F.);
#22865=ORIENTED_EDGE('',*,*,#16125,.F.);
#22866=ORIENTED_EDGE('',*,*,#16120,.F.);
#22867=ORIENTED_EDGE('',*,*,#16112,.F.);
#22868=ORIENTED_EDGE('',*,*,#16127,.F.);
#22869=ORIENTED_EDGE('',*,*,#16128,.F.);
#22870=ORIENTED_EDGE('',*,*,#16129,.F.);
#22871=ORIENTED_EDGE('',*,*,#16130,.F.);
#22872=ORIENTED_EDGE('',*,*,#16131,.F.);
#22873=ORIENTED_EDGE('',*,*,#16132,.F.);
#22874=ORIENTED_EDGE('',*,*,#16133,.F.);
#22875=ORIENTED_EDGE('',*,*,#16134,.F.);
#22876=ORIENTED_EDGE('',*,*,#16135,.F.);
#22877=ORIENTED_EDGE('',*,*,#16136,.F.);
#22878=ORIENTED_EDGE('',*,*,#16137,.T.);
#22879=ORIENTED_EDGE('',*,*,#16134,.T.);
#22880=ORIENTED_EDGE('',*,*,#16137,.F.);
#22881=ORIENTED_EDGE('',*,*,#16138,.T.);
#22882=ORIENTED_EDGE('',*,*,#16139,.T.);
#22883=ORIENTED_EDGE('',*,*,#16140,.T.);
#22884=ORIENTED_EDGE('',*,*,#16139,.F.);
#22885=ORIENTED_EDGE('',*,*,#16141,.T.);
#22886=ORIENTED_EDGE('',*,*,#16140,.F.);
#22887=ORIENTED_EDGE('',*,*,#16141,.F.);
#22888=ORIENTED_EDGE('',*,*,#16142,.T.);
#22889=ORIENTED_EDGE('',*,*,#16143,.T.);
#22890=ORIENTED_EDGE('',*,*,#16142,.F.);
#22891=ORIENTED_EDGE('',*,*,#16144,.F.);
#22892=ORIENTED_EDGE('',*,*,#16127,.T.);
#22893=ORIENTED_EDGE('',*,*,#16143,.F.);
#22894=ORIENTED_EDGE('',*,*,#16145,.F.);
#22895=ORIENTED_EDGE('',*,*,#16146,.F.);
#22896=ORIENTED_EDGE('',*,*,#16147,.F.);
#22897=ORIENTED_EDGE('',*,*,#16148,.F.);
#22898=ORIENTED_EDGE('',*,*,#16149,.F.);
#22899=ORIENTED_EDGE('',*,*,#16138,.F.);
#22900=ORIENTED_EDGE('',*,*,#16149,.T.);
#22901=ORIENTED_EDGE('',*,*,#16150,.T.);
#22902=ORIENTED_EDGE('',*,*,#16151,.T.);
#22903=ORIENTED_EDGE('',*,*,#16152,.T.);
#22904=ORIENTED_EDGE('',*,*,#16153,.T.);
#22905=ORIENTED_EDGE('',*,*,#16154,.T.);
#22906=ORIENTED_EDGE('',*,*,#16130,.T.);
#22907=ORIENTED_EDGE('',*,*,#16155,.T.);
#22908=ORIENTED_EDGE('',*,*,#16155,.F.);
#22909=ORIENTED_EDGE('',*,*,#16129,.T.);
#22910=ORIENTED_EDGE('',*,*,#16156,.T.);
#22911=ORIENTED_EDGE('',*,*,#16145,.T.);
#22912=ORIENTED_EDGE('',*,*,#16147,.T.);
#22913=ORIENTED_EDGE('',*,*,#16157,.F.);
#22914=ORIENTED_EDGE('',*,*,#16158,.F.);
#22915=ORIENTED_EDGE('',*,*,#16159,.F.);
#22916=ORIENTED_EDGE('',*,*,#16160,.F.);
#22917=ORIENTED_EDGE('',*,*,#16161,.F.);
#22918=ORIENTED_EDGE('',*,*,#16162,.F.);
#22919=ORIENTED_EDGE('',*,*,#16163,.F.);
#22920=ORIENTED_EDGE('',*,*,#16164,.F.);
#22921=ORIENTED_EDGE('',*,*,#16165,.F.);
#22922=ORIENTED_EDGE('',*,*,#16132,.T.);
#22923=ORIENTED_EDGE('',*,*,#16166,.T.);
#22924=ORIENTED_EDGE('',*,*,#16167,.T.);
#22925=ORIENTED_EDGE('',*,*,#16168,.T.);
#22926=ORIENTED_EDGE('',*,*,#16169,.T.);
#22927=ORIENTED_EDGE('',*,*,#16170,.T.);
#22928=ORIENTED_EDGE('',*,*,#16166,.F.);
#22929=ORIENTED_EDGE('',*,*,#16131,.T.);
#22930=ORIENTED_EDGE('',*,*,#16154,.F.);
#22931=ORIENTED_EDGE('',*,*,#16171,.F.);
#22932=ORIENTED_EDGE('',*,*,#16148,.T.);
#22933=ORIENTED_EDGE('',*,*,#16170,.F.);
#22934=ORIENTED_EDGE('',*,*,#16172,.F.);
#22935=ORIENTED_EDGE('',*,*,#16150,.F.);
#22936=ORIENTED_EDGE('',*,*,#16173,.T.);
#22937=ORIENTED_EDGE('',*,*,#16174,.T.);
#22938=ORIENTED_EDGE('',*,*,#16175,.T.);
#22939=ORIENTED_EDGE('',*,*,#16176,.T.);
#22940=ORIENTED_EDGE('',*,*,#16177,.T.);
#22941=ORIENTED_EDGE('',*,*,#16178,.T.);
#22942=ORIENTED_EDGE('',*,*,#16179,.F.);
#22943=ORIENTED_EDGE('',*,*,#16180,.F.);
#22944=ORIENTED_EDGE('',*,*,#16181,.F.);
#22945=ORIENTED_EDGE('',*,*,#16178,.F.);
#22946=ORIENTED_EDGE('',*,*,#16172,.T.);
#22947=ORIENTED_EDGE('',*,*,#16169,.F.);
#22948=ORIENTED_EDGE('',*,*,#16182,.T.);
#22949=ORIENTED_EDGE('',*,*,#16151,.F.);
#22950=ORIENTED_EDGE('',*,*,#16171,.T.);
#22951=ORIENTED_EDGE('',*,*,#16153,.F.);
#22952=ORIENTED_EDGE('',*,*,#16183,.T.);
#22953=ORIENTED_EDGE('',*,*,#16167,.F.);
#22954=ORIENTED_EDGE('',*,*,#16168,.F.);
#22955=ORIENTED_EDGE('',*,*,#16183,.F.);
#22956=ORIENTED_EDGE('',*,*,#16152,.F.);
#22957=ORIENTED_EDGE('',*,*,#16182,.F.);
#22958=ORIENTED_EDGE('',*,*,#16177,.F.);
#22959=ORIENTED_EDGE('',*,*,#16184,.F.);
#22960=ORIENTED_EDGE('',*,*,#16185,.F.);
#22961=ORIENTED_EDGE('',*,*,#16164,.T.);
#22962=ORIENTED_EDGE('',*,*,#16186,.F.);
#22963=ORIENTED_EDGE('',*,*,#16187,.F.);
#22964=ORIENTED_EDGE('',*,*,#16188,.F.);
#22965=ORIENTED_EDGE('',*,*,#16160,.T.);
#22966=ORIENTED_EDGE('',*,*,#16189,.F.);
#22967=ORIENTED_EDGE('',*,*,#16158,.T.);
#22968=ORIENTED_EDGE('',*,*,#16190,.F.);
#22969=ORIENTED_EDGE('',*,*,#16191,.F.);
#22970=ORIENTED_EDGE('',*,*,#16192,.F.);
#22971=ORIENTED_EDGE('',*,*,#16193,.F.);
#22972=ORIENTED_EDGE('',*,*,#16186,.T.);
#22973=ORIENTED_EDGE('',*,*,#16163,.T.);
#22974=ORIENTED_EDGE('',*,*,#16194,.T.);
#22975=ORIENTED_EDGE('',*,*,#16192,.T.);
#22976=ORIENTED_EDGE('',*,*,#16195,.F.);
#22977=ORIENTED_EDGE('',*,*,#16189,.T.);
#22978=ORIENTED_EDGE('',*,*,#16159,.T.);
#22979=ORIENTED_EDGE('',*,*,#16162,.T.);
#22980=ORIENTED_EDGE('',*,*,#16196,.F.);
#22981=ORIENTED_EDGE('',*,*,#16197,.F.);
#22982=ORIENTED_EDGE('',*,*,#16194,.F.);
#22983=ORIENTED_EDGE('',*,*,#16187,.T.);
#22984=ORIENTED_EDGE('',*,*,#16195,.T.);
#22985=ORIENTED_EDGE('',*,*,#16191,.T.);
#22986=ORIENTED_EDGE('',*,*,#16198,.F.);
#22987=ORIENTED_EDGE('',*,*,#16184,.T.);
#22988=ORIENTED_EDGE('',*,*,#16193,.T.);
#22989=ORIENTED_EDGE('',*,*,#16197,.T.);
#22990=ORIENTED_EDGE('',*,*,#16199,.F.);
#22991=ORIENTED_EDGE('',*,*,#16156,.F.);
#22992=ORIENTED_EDGE('',*,*,#16133,.T.);
#22993=ORIENTED_EDGE('',*,*,#16165,.T.);
#22994=ORIENTED_EDGE('',*,*,#16185,.T.);
#22995=ORIENTED_EDGE('',*,*,#16199,.T.);
#22996=ORIENTED_EDGE('',*,*,#16196,.T.);
#22997=ORIENTED_EDGE('',*,*,#16161,.T.);
#22998=ORIENTED_EDGE('',*,*,#16188,.T.);
#22999=ORIENTED_EDGE('',*,*,#16198,.T.);
#23000=ORIENTED_EDGE('',*,*,#16190,.T.);
#23001=ORIENTED_EDGE('',*,*,#16157,.T.);
#23002=ORIENTED_EDGE('',*,*,#16146,.T.);
#23003=ORIENTED_EDGE('',*,*,#16135,.T.);
#23004=ORIENTED_EDGE('',*,*,#16136,.T.);
#23005=ORIENTED_EDGE('',*,*,#16200,.T.);
#23006=ORIENTED_EDGE('',*,*,#16201,.T.);
#23007=ORIENTED_EDGE('',*,*,#16202,.T.);
#23008=ORIENTED_EDGE('',*,*,#16203,.T.);
#23009=ORIENTED_EDGE('',*,*,#16204,.T.);
#23010=ORIENTED_EDGE('',*,*,#16205,.T.);
#23011=ORIENTED_EDGE('',*,*,#16206,.T.);
#23012=ORIENTED_EDGE('',*,*,#16207,.T.);
#23013=ORIENTED_EDGE('',*,*,#16208,.T.);
#23014=ORIENTED_EDGE('',*,*,#16209,.T.);
#23015=ORIENTED_EDGE('',*,*,#16210,.T.);
#23016=ORIENTED_EDGE('',*,*,#16211,.T.);
#23017=ORIENTED_EDGE('',*,*,#16212,.T.);
#23018=ORIENTED_EDGE('',*,*,#16213,.T.);
#23019=ORIENTED_EDGE('',*,*,#16214,.T.);
#23020=ORIENTED_EDGE('',*,*,#16215,.T.);
#23021=ORIENTED_EDGE('',*,*,#16216,.T.);
#23022=ORIENTED_EDGE('',*,*,#16179,.T.);
#23023=ORIENTED_EDGE('',*,*,#16181,.T.);
#23024=ORIENTED_EDGE('',*,*,#16180,.T.);
#23025=ORIENTED_EDGE('',*,*,#16144,.T.);
#23026=ORIENTED_EDGE('',*,*,#16128,.T.);
#23027=ORIENTED_EDGE('',*,*,#16217,.T.);
#23028=ORIENTED_EDGE('',*,*,#16218,.T.);
#23029=ORIENTED_EDGE('',*,*,#16219,.T.);
#23030=ORIENTED_EDGE('',*,*,#16220,.T.);
#23031=ORIENTED_EDGE('',*,*,#16221,.T.);
#23032=ORIENTED_EDGE('',*,*,#16222,.T.);
#23033=ORIENTED_EDGE('',*,*,#16223,.T.);
#23034=ORIENTED_EDGE('',*,*,#16224,.T.);
#23035=ORIENTED_EDGE('',*,*,#16225,.T.);
#23036=ORIENTED_EDGE('',*,*,#16226,.T.);
#23037=ORIENTED_EDGE('',*,*,#16227,.T.);
#23038=ORIENTED_EDGE('',*,*,#16228,.T.);
#23039=ORIENTED_EDGE('',*,*,#16229,.T.);
#23040=ORIENTED_EDGE('',*,*,#16230,.T.);
#23041=ORIENTED_EDGE('',*,*,#16231,.T.);
#23042=ORIENTED_EDGE('',*,*,#16232,.T.);
#23043=ORIENTED_EDGE('',*,*,#16233,.T.);
#23044=ORIENTED_EDGE('',*,*,#16234,.T.);
#23045=ORIENTED_EDGE('',*,*,#16235,.T.);
#23046=ORIENTED_EDGE('',*,*,#16236,.T.);
#23047=ORIENTED_EDGE('',*,*,#16237,.T.);
#23048=ORIENTED_EDGE('',*,*,#16238,.T.);
#23049=ORIENTED_EDGE('',*,*,#16239,.T.);
#23050=ORIENTED_EDGE('',*,*,#16240,.T.);
#23051=ORIENTED_EDGE('',*,*,#16241,.T.);
#23052=ORIENTED_EDGE('',*,*,#16242,.T.);
#23053=ORIENTED_EDGE('',*,*,#16243,.T.);
#23054=ORIENTED_EDGE('',*,*,#16244,.T.);
#23055=ORIENTED_EDGE('',*,*,#16245,.T.);
#23056=ORIENTED_EDGE('',*,*,#16246,.T.);
#23057=ORIENTED_EDGE('',*,*,#16247,.T.);
#23058=ORIENTED_EDGE('',*,*,#16211,.F.);
#23059=ORIENTED_EDGE('',*,*,#16248,.F.);
#23060=ORIENTED_EDGE('',*,*,#16246,.F.);
#23061=ORIENTED_EDGE('',*,*,#16249,.T.);
#23062=ORIENTED_EDGE('',*,*,#16210,.F.);
#23063=ORIENTED_EDGE('',*,*,#16250,.F.);
#23064=ORIENTED_EDGE('',*,*,#16247,.F.);
#23065=ORIENTED_EDGE('',*,*,#16248,.T.);
#23066=ORIENTED_EDGE('',*,*,#16212,.F.);
#23067=ORIENTED_EDGE('',*,*,#16249,.F.);
#23068=ORIENTED_EDGE('',*,*,#16245,.F.);
#23069=ORIENTED_EDGE('',*,*,#16251,.T.);
#23070=ORIENTED_EDGE('',*,*,#16213,.F.);
#23071=ORIENTED_EDGE('',*,*,#16251,.F.);
#23072=ORIENTED_EDGE('',*,*,#16244,.F.);
#23073=ORIENTED_EDGE('',*,*,#16252,.T.);
#23074=ORIENTED_EDGE('',*,*,#16214,.F.);
#23075=ORIENTED_EDGE('',*,*,#16252,.F.);
#23076=ORIENTED_EDGE('',*,*,#16243,.F.);
#23077=ORIENTED_EDGE('',*,*,#16253,.T.);
#23078=ORIENTED_EDGE('',*,*,#16215,.F.);
#23079=ORIENTED_EDGE('',*,*,#16253,.F.);
#23080=ORIENTED_EDGE('',*,*,#16242,.F.);
#23081=ORIENTED_EDGE('',*,*,#16254,.T.);
#23082=ORIENTED_EDGE('',*,*,#16216,.F.);
#23083=ORIENTED_EDGE('',*,*,#16254,.F.);
#23084=ORIENTED_EDGE('',*,*,#16241,.F.);
#23085=ORIENTED_EDGE('',*,*,#16255,.T.);
#23086=ORIENTED_EDGE('',*,*,#16209,.F.);
#23087=ORIENTED_EDGE('',*,*,#16255,.F.);
#23088=ORIENTED_EDGE('',*,*,#16240,.F.);
#23089=ORIENTED_EDGE('',*,*,#16250,.T.);
#23090=ORIENTED_EDGE('',*,*,#16225,.F.);
#23091=ORIENTED_EDGE('',*,*,#16256,.F.);
#23092=ORIENTED_EDGE('',*,*,#16257,.F.);
#23093=ORIENTED_EDGE('',*,*,#16258,.T.);
#23094=ORIENTED_EDGE('',*,*,#16224,.F.);
#23095=ORIENTED_EDGE('',*,*,#16259,.F.);
#23096=ORIENTED_EDGE('',*,*,#16260,.F.);
#23097=ORIENTED_EDGE('',*,*,#16256,.T.);
#23098=ORIENTED_EDGE('',*,*,#16223,.F.);
#23099=ORIENTED_EDGE('',*,*,#16261,.F.);
#23100=ORIENTED_EDGE('',*,*,#16262,.F.);
#23101=ORIENTED_EDGE('',*,*,#16259,.T.);
#23102=ORIENTED_EDGE('',*,*,#16232,.F.);
#23103=ORIENTED_EDGE('',*,*,#16263,.F.);
#23104=ORIENTED_EDGE('',*,*,#16264,.F.);
#23105=ORIENTED_EDGE('',*,*,#16265,.T.);
#23106=ORIENTED_EDGE('',*,*,#16231,.F.);
#23107=ORIENTED_EDGE('',*,*,#16266,.F.);
#23108=ORIENTED_EDGE('',*,*,#16267,.F.);
#23109=ORIENTED_EDGE('',*,*,#16263,.T.);
#23110=ORIENTED_EDGE('',*,*,#16230,.F.);
#23111=ORIENTED_EDGE('',*,*,#16268,.F.);
#23112=ORIENTED_EDGE('',*,*,#16269,.F.);
#23113=ORIENTED_EDGE('',*,*,#16266,.T.);
#23114=ORIENTED_EDGE('',*,*,#16229,.F.);
#23115=ORIENTED_EDGE('',*,*,#16270,.F.);
#23116=ORIENTED_EDGE('',*,*,#16271,.F.);
#23117=ORIENTED_EDGE('',*,*,#16268,.T.);
#23118=ORIENTED_EDGE('',*,*,#16228,.F.);
#23119=ORIENTED_EDGE('',*,*,#16272,.F.);
#23120=ORIENTED_EDGE('',*,*,#16273,.F.);
#23121=ORIENTED_EDGE('',*,*,#16270,.T.);
#23122=ORIENTED_EDGE('',*,*,#16227,.F.);
#23123=ORIENTED_EDGE('',*,*,#16274,.F.);
#23124=ORIENTED_EDGE('',*,*,#16275,.F.);
#23125=ORIENTED_EDGE('',*,*,#16272,.T.);
#23126=ORIENTED_EDGE('',*,*,#16226,.F.);
#23127=ORIENTED_EDGE('',*,*,#16258,.F.);
#23128=ORIENTED_EDGE('',*,*,#16276,.F.);
#23129=ORIENTED_EDGE('',*,*,#16274,.T.);
#23130=ORIENTED_EDGE('',*,*,#16233,.F.);
#23131=ORIENTED_EDGE('',*,*,#16265,.F.);
#23132=ORIENTED_EDGE('',*,*,#16277,.F.);
#23133=ORIENTED_EDGE('',*,*,#16261,.T.);
#23134=ORIENTED_EDGE('',*,*,#16262,.T.);
#23135=ORIENTED_EDGE('',*,*,#16277,.T.);
#23136=ORIENTED_EDGE('',*,*,#16264,.T.);
#23137=ORIENTED_EDGE('',*,*,#16267,.T.);
#23138=ORIENTED_EDGE('',*,*,#16269,.T.);
#23139=ORIENTED_EDGE('',*,*,#16271,.T.);
#23140=ORIENTED_EDGE('',*,*,#16273,.T.);
#23141=ORIENTED_EDGE('',*,*,#16275,.T.);
#23142=ORIENTED_EDGE('',*,*,#16276,.T.);
#23143=ORIENTED_EDGE('',*,*,#16257,.T.);
#23144=ORIENTED_EDGE('',*,*,#16260,.T.);
#23145=ORIENTED_EDGE('',*,*,#16278,.T.);
#23146=ORIENTED_EDGE('',*,*,#16279,.T.);
#23147=ORIENTED_EDGE('',*,*,#16280,.T.);
#23148=ORIENTED_EDGE('',*,*,#16281,.T.);
#23149=ORIENTED_EDGE('',*,*,#16282,.T.);
#23150=ORIENTED_EDGE('',*,*,#16283,.T.);
#23151=ORIENTED_EDGE('',*,*,#16219,.F.);
#23152=ORIENTED_EDGE('',*,*,#16284,.F.);
#23153=ORIENTED_EDGE('',*,*,#16280,.F.);
#23154=ORIENTED_EDGE('',*,*,#16285,.T.);
#23155=ORIENTED_EDGE('',*,*,#16218,.F.);
#23156=ORIENTED_EDGE('',*,*,#16286,.F.);
#23157=ORIENTED_EDGE('',*,*,#16281,.F.);
#23158=ORIENTED_EDGE('',*,*,#16284,.T.);
#23159=ORIENTED_EDGE('',*,*,#16220,.F.);
#23160=ORIENTED_EDGE('',*,*,#16285,.F.);
#23161=ORIENTED_EDGE('',*,*,#16279,.F.);
#23162=ORIENTED_EDGE('',*,*,#16287,.T.);
#23163=ORIENTED_EDGE('',*,*,#16221,.F.);
#23164=ORIENTED_EDGE('',*,*,#16287,.F.);
#23165=ORIENTED_EDGE('',*,*,#16278,.F.);
#23166=ORIENTED_EDGE('',*,*,#16288,.T.);
#23167=ORIENTED_EDGE('',*,*,#16222,.F.);
#23168=ORIENTED_EDGE('',*,*,#16288,.F.);
#23169=ORIENTED_EDGE('',*,*,#16283,.F.);
#23170=ORIENTED_EDGE('',*,*,#16289,.T.);
#23171=ORIENTED_EDGE('',*,*,#16217,.F.);
#23172=ORIENTED_EDGE('',*,*,#16289,.F.);
#23173=ORIENTED_EDGE('',*,*,#16282,.F.);
#23174=ORIENTED_EDGE('',*,*,#16286,.T.);
#23175=ORIENTED_EDGE('',*,*,#16238,.F.);
#23176=ORIENTED_EDGE('',*,*,#16290,.F.);
#23177=ORIENTED_EDGE('',*,*,#16291,.F.);
#23178=ORIENTED_EDGE('',*,*,#16292,.T.);
#23179=ORIENTED_EDGE('',*,*,#16237,.F.);
#23180=ORIENTED_EDGE('',*,*,#16293,.F.);
#23181=ORIENTED_EDGE('',*,*,#16294,.F.);
#23182=ORIENTED_EDGE('',*,*,#16290,.T.);
#23183=ORIENTED_EDGE('',*,*,#16236,.F.);
#23184=ORIENTED_EDGE('',*,*,#16295,.F.);
#23185=ORIENTED_EDGE('',*,*,#16296,.F.);
#23186=ORIENTED_EDGE('',*,*,#16293,.T.);
#23187=ORIENTED_EDGE('',*,*,#16235,.F.);
#23188=ORIENTED_EDGE('',*,*,#16297,.F.);
#23189=ORIENTED_EDGE('',*,*,#16298,.F.);
#23190=ORIENTED_EDGE('',*,*,#16295,.T.);
#23191=ORIENTED_EDGE('',*,*,#16239,.F.);
#23192=ORIENTED_EDGE('',*,*,#16292,.F.);
#23193=ORIENTED_EDGE('',*,*,#16299,.F.);
#23194=ORIENTED_EDGE('',*,*,#16300,.T.);
#23195=ORIENTED_EDGE('',*,*,#16234,.F.);
#23196=ORIENTED_EDGE('',*,*,#16300,.F.);
#23197=ORIENTED_EDGE('',*,*,#16301,.F.);
#23198=ORIENTED_EDGE('',*,*,#16297,.T.);
#23199=ORIENTED_EDGE('',*,*,#16296,.T.);
#23200=ORIENTED_EDGE('',*,*,#16298,.T.);
#23201=ORIENTED_EDGE('',*,*,#16301,.T.);
#23202=ORIENTED_EDGE('',*,*,#16299,.T.);
#23203=ORIENTED_EDGE('',*,*,#16291,.T.);
#23204=ORIENTED_EDGE('',*,*,#16294,.T.);
#23205=ORIENTED_EDGE('',*,*,#16203,.F.);
#23206=ORIENTED_EDGE('',*,*,#16302,.F.);
#23207=ORIENTED_EDGE('',*,*,#16303,.F.);
#23208=ORIENTED_EDGE('',*,*,#16304,.T.);
#23209=ORIENTED_EDGE('',*,*,#16202,.F.);
#23210=ORIENTED_EDGE('',*,*,#16305,.F.);
#23211=ORIENTED_EDGE('',*,*,#16306,.F.);
#23212=ORIENTED_EDGE('',*,*,#16302,.T.);
#23213=ORIENTED_EDGE('',*,*,#16201,.F.);
#23214=ORIENTED_EDGE('',*,*,#16307,.F.);
#23215=ORIENTED_EDGE('',*,*,#16308,.F.);
#23216=ORIENTED_EDGE('',*,*,#16305,.T.);
#23217=ORIENTED_EDGE('',*,*,#16200,.F.);
#23218=ORIENTED_EDGE('',*,*,#16309,.F.);
#23219=ORIENTED_EDGE('',*,*,#16310,.F.);
#23220=ORIENTED_EDGE('',*,*,#16307,.T.);
#23221=ORIENTED_EDGE('',*,*,#16208,.F.);
#23222=ORIENTED_EDGE('',*,*,#16311,.F.);
#23223=ORIENTED_EDGE('',*,*,#16312,.F.);
#23224=ORIENTED_EDGE('',*,*,#16309,.T.);
#23225=ORIENTED_EDGE('',*,*,#16176,.F.);
#23226=ORIENTED_EDGE('',*,*,#16313,.F.);
#23227=ORIENTED_EDGE('',*,*,#16314,.F.);
#23228=ORIENTED_EDGE('',*,*,#16315,.T.);
#23229=ORIENTED_EDGE('',*,*,#16175,.F.);
#23230=ORIENTED_EDGE('',*,*,#16316,.F.);
#23231=ORIENTED_EDGE('',*,*,#16317,.F.);
#23232=ORIENTED_EDGE('',*,*,#16313,.T.);
#23233=ORIENTED_EDGE('',*,*,#16207,.F.);
#23234=ORIENTED_EDGE('',*,*,#16318,.F.);
#23235=ORIENTED_EDGE('',*,*,#16319,.F.);
#23236=ORIENTED_EDGE('',*,*,#16311,.T.);
#23237=ORIENTED_EDGE('',*,*,#16206,.F.);
#23238=ORIENTED_EDGE('',*,*,#16320,.F.);
#23239=ORIENTED_EDGE('',*,*,#16321,.F.);
#23240=ORIENTED_EDGE('',*,*,#16318,.T.);
#23241=ORIENTED_EDGE('',*,*,#16205,.F.);
#23242=ORIENTED_EDGE('',*,*,#16322,.F.);
#23243=ORIENTED_EDGE('',*,*,#16323,.F.);
#23244=ORIENTED_EDGE('',*,*,#16320,.T.);
#23245=ORIENTED_EDGE('',*,*,#16204,.F.);
#23246=ORIENTED_EDGE('',*,*,#16304,.F.);
#23247=ORIENTED_EDGE('',*,*,#16324,.F.);
#23248=ORIENTED_EDGE('',*,*,#16322,.T.);
#23249=ORIENTED_EDGE('',*,*,#16174,.F.);
#23250=ORIENTED_EDGE('',*,*,#16325,.F.);
#23251=ORIENTED_EDGE('',*,*,#16326,.F.);
#23252=ORIENTED_EDGE('',*,*,#16316,.T.);
#23253=ORIENTED_EDGE('',*,*,#16173,.F.);
#23254=ORIENTED_EDGE('',*,*,#16315,.F.);
#23255=ORIENTED_EDGE('',*,*,#16327,.F.);
#23256=ORIENTED_EDGE('',*,*,#16325,.T.);
#23257=ORIENTED_EDGE('',*,*,#16310,.T.);
#23258=ORIENTED_EDGE('',*,*,#16312,.T.);
#23259=ORIENTED_EDGE('',*,*,#16319,.T.);
#23260=ORIENTED_EDGE('',*,*,#16321,.T.);
#23261=ORIENTED_EDGE('',*,*,#16323,.T.);
#23262=ORIENTED_EDGE('',*,*,#16324,.T.);
#23263=ORIENTED_EDGE('',*,*,#16303,.T.);
#23264=ORIENTED_EDGE('',*,*,#16306,.T.);
#23265=ORIENTED_EDGE('',*,*,#16308,.T.);
#23266=ORIENTED_EDGE('',*,*,#16317,.T.);
#23267=ORIENTED_EDGE('',*,*,#16326,.T.);
#23268=ORIENTED_EDGE('',*,*,#16327,.T.);
#23269=ORIENTED_EDGE('',*,*,#16314,.T.);
#24148=CYLINDRICAL_SURFACE('',#28282,17.5);
#24149=CYLINDRICAL_SURFACE('',#28284,17.5);
#24150=CYLINDRICAL_SURFACE('',#28286,13.);
#24151=CYLINDRICAL_SURFACE('',#28288,13.);
#24152=CYLINDRICAL_SURFACE('',#28290,13.);
#24153=CYLINDRICAL_SURFACE('',#28292,13.);
#24154=CYLINDRICAL_SURFACE('',#28294,27.5);
#24155=CYLINDRICAL_SURFACE('',#28298,9.5);
#24156=CYLINDRICAL_SURFACE('',#28301,2.5);
#24157=CYLINDRICAL_SURFACE('',#28306,3.3);
#24158=CYLINDRICAL_SURFACE('',#28310,2.5);
#24159=CYLINDRICAL_SURFACE('',#28314,5.5);
#24160=CYLINDRICAL_SURFACE('',#28315,5.5);
#24161=CYLINDRICAL_SURFACE('',#28319,2.5);
#24162=CYLINDRICAL_SURFACE('',#28320,2.5);
#24163=CYLINDRICAL_SURFACE('',#28325,3.3);
#24164=CYLINDRICAL_SURFACE('',#28347,9.5);
#24165=CYLINDRICAL_SURFACE('',#28348,9.5);
#24166=CYLINDRICAL_SURFACE('',#28349,27.5);
#24167=CYLINDRICAL_SURFACE('',#28351,2.1);
#24168=CYLINDRICAL_SURFACE('',#28356,13.);
#24169=CYLINDRICAL_SURFACE('',#28358,13.);
#24170=CYLINDRICAL_SURFACE('',#28360,13.);
#24171=CYLINDRICAL_SURFACE('',#28362,17.5);
#24172=CYLINDRICAL_SURFACE('',#28364,17.5);
#24173=CYLINDRICAL_SURFACE('',#28366,13.);
#24174=CYLINDRICAL_SURFACE('',#28372,27.5);
#24175=CYLINDRICAL_SURFACE('',#28396,27.);
#24176=CYLINDRICAL_SURFACE('',#28427,27.);
#24177=CYLINDRICAL_SURFACE('',#28428,27.);
#24178=CYLINDRICAL_SURFACE('',#28449,27.);
#24179=CYLINDRICAL_SURFACE('',#28455,1.4361111111);
#24180=CYLINDRICAL_SURFACE('',#28466,0.4033333333);
#24181=CYLINDRICAL_SURFACE('',#28468,27.);
#25444=ADVANCED_FACE('',(#3491),#2148,.T.);
#25445=ADVANCED_FACE('',(#3492),#557,.T.);
#25446=ADVANCED_FACE('',(#3493),#2149,.T.);
#25447=ADVANCED_FACE('',(#3494),#2150,.T.);
#25448=ADVANCED_FACE('',(#3495),#24148,.F.);
#25449=ADVANCED_FACE('',(#3496),#24149,.F.);
#25450=ADVANCED_FACE('',(#3497),#24150,.F.);
#25451=ADVANCED_FACE('',(#3498),#24151,.F.);
#25452=ADVANCED_FACE('',(#3499),#24152,.F.);
#25453=ADVANCED_FACE('',(#3500),#24153,.F.);
#25454=ADVANCED_FACE('',(#3501,#1432,#1433),#24154,.T.);
#25455=ADVANCED_FACE('',(#3502),#24155,.F.);
#25456=ADVANCED_FACE('',(#3503),#2151,.F.);
#25457=ADVANCED_FACE('',(#3504),#24156,.F.);
#25458=ADVANCED_FACE('',(#3505,#1434),#2152,.F.);
#25459=ADVANCED_FACE('',(#3506),#24157,.F.);
#25460=ADVANCED_FACE('',(#3507,#1435),#2153,.F.);
#25461=ADVANCED_FACE('',(#3508),#24158,.F.);
#25462=ADVANCED_FACE('',(#3509,#1436),#2154,.T.);
#25463=ADVANCED_FACE('',(#3510,#1437),#2155,.T.);
#25464=ADVANCED_FACE('',(#3511),#24159,.F.);
#25465=ADVANCED_FACE('',(#3512),#24160,.F.);
#25466=ADVANCED_FACE('',(#3513,#1438),#2156,.T.);
#25467=ADVANCED_FACE('',(#3514),#24161,.F.);
#25468=ADVANCED_FACE('',(#3515),#24162,.F.);
#25469=ADVANCED_FACE('',(#3516,#1439),#2157,.F.);
#25470=ADVANCED_FACE('',(#3517),#24163,.F.);
#25471=ADVANCED_FACE('',(#3518,#1440),#2158,.F.);
#25472=ADVANCED_FACE('',(#3519,#1441),#2159,.T.);
#25473=ADVANCED_FACE('',(#3520),#2160,.T.);
#25474=ADVANCED_FACE('',(#3521),#558,.T.);
#25475=ADVANCED_FACE('',(#3522),#2161,.F.);
#25476=ADVANCED_FACE('',(#3523),#24164,.F.);
#25477=ADVANCED_FACE('',(#3524),#24165,.F.);
#25478=ADVANCED_FACE('',(#3525),#24166,.T.);
#25479=ADVANCED_FACE('',(#3526),#24167,.F.);
#25480=ADVANCED_FACE('',(#3527),#2162,.T.);
#25481=ADVANCED_FACE('',(#3528),#2163,.T.);
#25482=ADVANCED_FACE('',(#3529,#1442),#2164,.F.);
#25483=ADVANCED_FACE('',(#3530),#24168,.F.);
#25484=ADVANCED_FACE('',(#3531),#24169,.F.);
#25485=ADVANCED_FACE('',(#3532),#24170,.F.);
#25486=ADVANCED_FACE('',(#3533),#24171,.F.);
#25487=ADVANCED_FACE('',(#3534),#24172,.F.);
#25488=ADVANCED_FACE('',(#3535),#24173,.F.);
#25489=ADVANCED_FACE('',(#3536),#2165,.T.);
#25490=ADVANCED_FACE('',(#3537),#2166,.T.);
#25491=ADVANCED_FACE('',(#3538,#1443,#1444,#1445,#1446,#1447,#1448,#1449,
#1450),#24174,.T.);
#25492=ADVANCED_FACE('',(#3539),#24175,.T.);
#25493=ADVANCED_FACE('',(#3540),#2167,.F.);
#25494=ADVANCED_FACE('',(#3541),#2168,.F.);
#25495=ADVANCED_FACE('',(#3542),#2169,.F.);
#25496=ADVANCED_FACE('',(#3543),#2170,.F.);
#25497=ADVANCED_FACE('',(#3544),#2171,.F.);
#25498=ADVANCED_FACE('',(#3545),#2172,.F.);
#25499=ADVANCED_FACE('',(#3546),#2173,.F.);
#25500=ADVANCED_FACE('',(#3547),#2174,.F.);
#25501=ADVANCED_FACE('',(#3548),#2175,.F.);
#25502=ADVANCED_FACE('',(#3549),#2176,.F.);
#25503=ADVANCED_FACE('',(#3550),#2177,.F.);
#25504=ADVANCED_FACE('',(#3551),#2178,.F.);
#25505=ADVANCED_FACE('',(#3552),#2179,.F.);
#25506=ADVANCED_FACE('',(#3553),#2180,.F.);
#25507=ADVANCED_FACE('',(#3554),#2181,.F.);
#25508=ADVANCED_FACE('',(#3555),#2182,.F.);
#25509=ADVANCED_FACE('',(#3556),#2183,.F.);
#25510=ADVANCED_FACE('',(#3557),#2184,.F.);
#25511=ADVANCED_FACE('',(#3558),#2185,.F.);
#25512=ADVANCED_FACE('',(#3559),#24176,.T.);
#25513=ADVANCED_FACE('',(#3560),#24177,.T.);
#25514=ADVANCED_FACE('',(#3561),#2186,.F.);
#25515=ADVANCED_FACE('',(#3562),#2187,.F.);
#25516=ADVANCED_FACE('',(#3563),#2188,.F.);
#25517=ADVANCED_FACE('',(#3564),#2189,.F.);
#25518=ADVANCED_FACE('',(#3565),#2190,.F.);
#25519=ADVANCED_FACE('',(#3566),#2191,.F.);
#25520=ADVANCED_FACE('',(#3567),#2192,.F.);
#25521=ADVANCED_FACE('',(#3568),#2193,.F.);
#25522=ADVANCED_FACE('',(#3569),#2194,.F.);
#25523=ADVANCED_FACE('',(#3570),#2195,.F.);
#25524=ADVANCED_FACE('',(#3571),#2196,.F.);
#25525=ADVANCED_FACE('',(#3572),#2197,.F.);
#25526=ADVANCED_FACE('',(#3573),#24178,.T.);
#25527=ADVANCED_FACE('',(#3574),#2198,.F.);
#25528=ADVANCED_FACE('',(#3575),#2199,.F.);
#25529=ADVANCED_FACE('',(#3576),#2200,.F.);
#25530=ADVANCED_FACE('',(#3577),#24179,.F.);
#25531=ADVANCED_FACE('',(#3578),#2201,.F.);
#25532=ADVANCED_FACE('',(#3579),#2202,.T.);
#25533=ADVANCED_FACE('',(#3580),#2203,.T.);
#25534=ADVANCED_FACE('',(#3581),#2204,.F.);
#25535=ADVANCED_FACE('',(#3582),#2205,.F.);
#25536=ADVANCED_FACE('',(#3583),#2206,.F.);
#25537=ADVANCED_FACE('',(#3584),#2207,.F.);
#25538=ADVANCED_FACE('',(#3585),#24180,.T.);
#25539=ADVANCED_FACE('',(#3586),#2208,.T.);
#25540=ADVANCED_FACE('',(#3587,#1451),#24181,.T.);
#25690=CLOSED_SHELL('',(#25444,#25445,#25446,#25447,#25448,#25449,#25450,
#25451,#25452,#25453,#25454,#25455,#25456,#25457,#25458,#25459,#25460,#25461,
#25462,#25463,#25464));
#25691=CLOSED_SHELL('',(#25465,#25466,#25467,#25468,#25469,#25470,#25471,
#25472,#25473,#25474,#25475,#25476,#25477,#25478,#25479,#25480,#25481,#25482,
#25483,#25484,#25485,#25486,#25487,#25488,#25489,#25490,#25491,#25492,#25493,
#25494,#25495,#25496,#25497,#25498,#25499,#25500,#25501,#25502,#25503,#25504,
#25505,#25506,#25507,#25508,#25509,#25510,#25511,#25512,#25513,#25514,#25515,
#25516,#25517,#25518,#25519,#25520,#25521,#25522,#25523,#25524,#25525,#25526,
#25527,#25528,#25529,#25530,#25531,#25532,#25533,#25534,#25535,#25536,#25537,
#25538,#25539,#25540));
#28266=AXIS2_PLACEMENT_3D('',#65193,#34889,#34890);
#28267=AXIS2_PLACEMENT_3D('',#65194,#34891,#34892);
#28268=AXIS2_PLACEMENT_3D('',#65199,#34894,#34895);
#28269=AXIS2_PLACEMENT_3D('',#65202,#34897,#34898);
#28270=AXIS2_PLACEMENT_3D('',#65203,#34899,#34900);
#28271=AXIS2_PLACEMENT_3D('',#65206,#34901,#34902);
#28272=AXIS2_PLACEMENT_3D('',#65209,#34905,#34906);
#28273=AXIS2_PLACEMENT_3D('',#65212,#34907,#34908);
#28274=AXIS2_PLACEMENT_3D('',#65214,#34909,#34910);
#28275=AXIS2_PLACEMENT_3D('',#65216,#34911,#34912);
#28276=AXIS2_PLACEMENT_3D('',#65217,#34913,#34914);
#28277=AXIS2_PLACEMENT_3D('',#65218,#34915,#34916);
#28278=AXIS2_PLACEMENT_3D('',#65221,#34917,#34918);
#28279=AXIS2_PLACEMENT_3D('',#65223,#34919,#34920);
#28280=AXIS2_PLACEMENT_3D('',#65225,#34921,#34922);
#28281=AXIS2_PLACEMENT_3D('',#65226,#34923,#34924);
#28282=AXIS2_PLACEMENT_3D('',#65227,#34925,#34926);
#28283=AXIS2_PLACEMENT_3D('',#65230,#34927,#34928);
#28284=AXIS2_PLACEMENT_3D('',#65233,#34931,#34932);
#28285=AXIS2_PLACEMENT_3D('',#65238,#34935,#34936);
#28286=AXIS2_PLACEMENT_3D('',#65239,#34937,#34938);
#28287=AXIS2_PLACEMENT_3D('',#65242,#34940,#34941);
#28288=AXIS2_PLACEMENT_3D('',#65243,#34942,#34943);
#28289=AXIS2_PLACEMENT_3D('',#65246,#34945,#34946);
#28290=AXIS2_PLACEMENT_3D('',#65247,#34947,#34948);
#28291=AXIS2_PLACEMENT_3D('',#65249,#34949,#34950);
#28292=AXIS2_PLACEMENT_3D('',#65251,#34952,#34953);
#28293=AXIS2_PLACEMENT_3D('',#65253,#34954,#34955);
#28294=AXIS2_PLACEMENT_3D('',#65255,#34957,#34958);
#28295=AXIS2_PLACEMENT_3D('',#65256,#34959,#34960);
#28296=AXIS2_PLACEMENT_3D('',#65258,#34961,#34962);
#28297=AXIS2_PLACEMENT_3D('',#65262,#34965,#34966);
#28298=AXIS2_PLACEMENT_3D('',#65341,#34968,#34969);
#28299=AXIS2_PLACEMENT_3D('',#65345,#34971,#34972);
#28300=AXIS2_PLACEMENT_3D('',#65347,#34974,#34975);
#28301=AXIS2_PLACEMENT_3D('',#65350,#34978,#34979);
#28302=AXIS2_PLACEMENT_3D('',#65353,#34981,#34982);
#28303=AXIS2_PLACEMENT_3D('',#65354,#34983,#34984);
#28304=AXIS2_PLACEMENT_3D('',#65355,#34985,#34986);
#28305=AXIS2_PLACEMENT_3D('',#65357,#34987,#34988);
#28306=AXIS2_PLACEMENT_3D('',#65358,#34989,#34990);
#28307=AXIS2_PLACEMENT_3D('',#65360,#34991,#34992);
#28308=AXIS2_PLACEMENT_3D('',#65362,#34994,#34995);
#28309=AXIS2_PLACEMENT_3D('',#65364,#34996,#34997);
#28310=AXIS2_PLACEMENT_3D('',#65365,#34998,#34999);
#28311=AXIS2_PLACEMENT_3D('',#65367,#35000,#35001);
#28312=AXIS2_PLACEMENT_3D('',#65369,#35003,#35004);
#28313=AXIS2_PLACEMENT_3D('',#65370,#35005,#35006);
#28314=AXIS2_PLACEMENT_3D('',#65371,#35007,#35008);
#28315=AXIS2_PLACEMENT_3D('',#65372,#35009,#35010);
#28316=AXIS2_PLACEMENT_3D('',#65375,#35011,#35012);
#28317=AXIS2_PLACEMENT_3D('',#65406,#35013,#35014);
#28318=AXIS2_PLACEMENT_3D('',#65418,#35020,#35021);
#28319=AXIS2_PLACEMENT_3D('',#65419,#35022,#35023);
#28320=AXIS2_PLACEMENT_3D('',#65463,#35025,#35026);
#28321=AXIS2_PLACEMENT_3D('',#65465,#35027,#35028);
#28322=AXIS2_PLACEMENT_3D('',#65468,#35030,#35031);
#28323=AXIS2_PLACEMENT_3D('',#65469,#35032,#35033);
#28324=AXIS2_PLACEMENT_3D('',#65471,#35034,#35035);
#28325=AXIS2_PLACEMENT_3D('',#65472,#35036,#35037);
#28326=AXIS2_PLACEMENT_3D('',#65475,#35039,#35040);
#28327=AXIS2_PLACEMENT_3D('',#65476,#35041,#35042);
#28328=AXIS2_PLACEMENT_3D('',#65478,#35044,#35045);
#28329=AXIS2_PLACEMENT_3D('',#65489,#35051,#35052);
#28330=AXIS2_PLACEMENT_3D('',#65491,#35053,#35054);
#28331=AXIS2_PLACEMENT_3D('',#65498,#35058,#35059);
#28332=AXIS2_PLACEMENT_3D('',#65499,#35060,#35061);
#28333=AXIS2_PLACEMENT_3D('',#65500,#35062,#35063);
#28334=AXIS2_PLACEMENT_3D('',#65501,#35064,#35065);
#28335=AXIS2_PLACEMENT_3D('',#65502,#35066,#35067);
#28336=AXIS2_PLACEMENT_3D('',#65504,#35068,#35069);
#28337=AXIS2_PLACEMENT_3D('',#65506,#35070,#35071);
#28338=AXIS2_PLACEMENT_3D('',#65508,#35072,#35073);
#28339=AXIS2_PLACEMENT_3D('',#65510,#35074,#35075);
#28340=AXIS2_PLACEMENT_3D('',#65512,#35076,#35077);
#28341=AXIS2_PLACEMENT_3D('',#65514,#35078,#35079);
#28342=AXIS2_PLACEMENT_3D('',#65516,#35080,#35081);
#28343=AXIS2_PLACEMENT_3D('',#65518,#35082,#35083);
#28344=AXIS2_PLACEMENT_3D('',#65519,#35084,#35085);
#28345=AXIS2_PLACEMENT_3D('',#65521,#35086,#35087);
#28346=AXIS2_PLACEMENT_3D('',#65528,#35091,#35092);
#28347=AXIS2_PLACEMENT_3D('',#65529,#35093,#35094);
#28348=AXIS2_PLACEMENT_3D('',#65531,#35096,#35097);
#28349=AXIS2_PLACEMENT_3D('',#65533,#35099,#35100);
#28350=AXIS2_PLACEMENT_3D('',#65558,#35103,#35104);
#28351=AXIS2_PLACEMENT_3D('',#65559,#35105,#35106);
#28352=AXIS2_PLACEMENT_3D('',#65561,#35107,#35108);
#28353=AXIS2_PLACEMENT_3D('',#65655,#35110,#35111);
#28354=AXIS2_PLACEMENT_3D('',#65657,#35113,#35114);
#28355=AXIS2_PLACEMENT_3D('',#65659,#35116,#35117);
#28356=AXIS2_PLACEMENT_3D('',#65660,#35118,#35119);
#28357=AXIS2_PLACEMENT_3D('',#65663,#35120,#35121);
#28358=AXIS2_PLACEMENT_3D('',#65666,#35124,#35125);
#28359=AXIS2_PLACEMENT_3D('',#65669,#35126,#35127);
#28360=AXIS2_PLACEMENT_3D('',#65672,#35130,#35131);
#28361=AXIS2_PLACEMENT_3D('',#65676,#35133,#35134);
#28362=AXIS2_PLACEMENT_3D('',#65678,#35136,#35137);
#28363=AXIS2_PLACEMENT_3D('',#65680,#35138,#35139);
#28364=AXIS2_PLACEMENT_3D('',#65682,#35141,#35142);
#28365=AXIS2_PLACEMENT_3D('',#65683,#35143,#35144);
#28366=AXIS2_PLACEMENT_3D('',#65684,#35145,#35146);
#28367=AXIS2_PLACEMENT_3D('',#65687,#35148,#35149);
#28368=AXIS2_PLACEMENT_3D('',#65688,#35150,#35151);
#28369=AXIS2_PLACEMENT_3D('',#65689,#35152,#35153);
#28370=AXIS2_PLACEMENT_3D('',#65690,#35154,#35155);
#28371=AXIS2_PLACEMENT_3D('',#65691,#35156,#35157);
#28372=AXIS2_PLACEMENT_3D('',#65692,#35158,#35159);
#28373=AXIS2_PLACEMENT_3D('',#65712,#35160,#35161);
#28374=AXIS2_PLACEMENT_3D('',#65716,#35163,#35164);
#28375=AXIS2_PLACEMENT_3D('',#65720,#35166,#35167);
#28376=AXIS2_PLACEMENT_3D('',#65724,#35169,#35170);
#28377=AXIS2_PLACEMENT_3D('',#65728,#35172,#35173);
#28378=AXIS2_PLACEMENT_3D('',#65732,#35175,#35176);
#28379=AXIS2_PLACEMENT_3D('',#65736,#35178,#35179);
#28380=AXIS2_PLACEMENT_3D('',#65740,#35181,#35182);
#28381=AXIS2_PLACEMENT_3D('',#65746,#35185,#35186);
#28382=AXIS2_PLACEMENT_3D('',#65748,#35187,#35188);
#28383=AXIS2_PLACEMENT_3D('',#65752,#35190,#35191);
#28384=AXIS2_PLACEMENT_3D('',#65753,#35192,#35193);
#28385=AXIS2_PLACEMENT_3D('',#65756,#35194,#35195);
#28386=AXIS2_PLACEMENT_3D('',#65760,#35197,#35198);
#28387=AXIS2_PLACEMENT_3D('',#65762,#35199,#35200);
#28388=AXIS2_PLACEMENT_3D('',#65766,#35202,#35203);
#28389=AXIS2_PLACEMENT_3D('',#65770,#35205,#35206);
#28390=AXIS2_PLACEMENT_3D('',#65772,#35207,#35208);
#28391=AXIS2_PLACEMENT_3D('',#65775,#35210,#35211);
#28392=AXIS2_PLACEMENT_3D('',#65778,#35212,#35213);
#28393=AXIS2_PLACEMENT_3D('',#65782,#35215,#35216);
#28394=AXIS2_PLACEMENT_3D('',#65784,#35217,#35218);
#28395=AXIS2_PLACEMENT_3D('',#65787,#35220,#35221);
#28396=AXIS2_PLACEMENT_3D('',#65788,#35222,#35223);
#28397=AXIS2_PLACEMENT_3D('',#65791,#35224,#35225);
#28398=AXIS2_PLACEMENT_3D('',#65795,#35227,#35228);
#28399=AXIS2_PLACEMENT_3D('',#65799,#35230,#35231);
#28400=AXIS2_PLACEMENT_3D('',#65803,#35233,#35234);
#28401=AXIS2_PLACEMENT_3D('',#65805,#35236,#35237);
#28402=AXIS2_PLACEMENT_3D('',#65808,#35240,#35241);
#28403=AXIS2_PLACEMENT_3D('',#65810,#35243,#35244);
#28404=AXIS2_PLACEMENT_3D('',#65812,#35246,#35247);
#28405=AXIS2_PLACEMENT_3D('',#65814,#35249,#35250);
#28406=AXIS2_PLACEMENT_3D('',#65816,#35252,#35253);
#28407=AXIS2_PLACEMENT_3D('',#65818,#35255,#35256);
#28408=AXIS2_PLACEMENT_3D('',#65820,#35258,#35259);
#28409=AXIS2_PLACEMENT_3D('',#65821,#35260,#35261);
#28410=AXIS2_PLACEMENT_3D('',#65825,#35263,#35264);
#28411=AXIS2_PLACEMENT_3D('',#65827,#35266,#35267);
#28412=AXIS2_PLACEMENT_3D('',#65831,#35270,#35271);
#28413=AXIS2_PLACEMENT_3D('',#65834,#35273,#35274);
#28414=AXIS2_PLACEMENT_3D('',#65835,#35275,#35276);
#28415=AXIS2_PLACEMENT_3D('',#65841,#35280,#35281);
#28416=AXIS2_PLACEMENT_3D('',#65844,#35283,#35284);
#28417=AXIS2_PLACEMENT_3D('',#65845,#35285,#35286);
#28418=AXIS2_PLACEMENT_3D('',#65848,#35288,#35289);
#28419=AXIS2_PLACEMENT_3D('',#65849,#35290,#35291);
#28420=AXIS2_PLACEMENT_3D('',#65853,#35294,#35295);
#28421=AXIS2_PLACEMENT_3D('',#65856,#35297,#35298);
#28422=AXIS2_PLACEMENT_3D('',#65857,#35299,#35300);
#28423=AXIS2_PLACEMENT_3D('',#65861,#35303,#35304);
#28424=AXIS2_PLACEMENT_3D('',#65862,#35305,#35306);
#28425=AXIS2_PLACEMENT_3D('',#65863,#35307,#35308);
#28426=AXIS2_PLACEMENT_3D('',#65864,#35309,#35310);
#28427=AXIS2_PLACEMENT_3D('',#65865,#35311,#35312);
#28428=AXIS2_PLACEMENT_3D('',#65866,#35313,#35314);
#28429=AXIS2_PLACEMENT_3D('',#65869,#35315,#35316);
#28430=AXIS2_PLACEMENT_3D('',#65873,#35318,#35319);
#28431=AXIS2_PLACEMENT_3D('',#65875,#35320,#35321);
#28432=AXIS2_PLACEMENT_3D('',#65878,#35323,#35324);
#28433=AXIS2_PLACEMENT_3D('',#65879,#35325,#35326);
#28434=AXIS2_PLACEMENT_3D('',#65882,#35329,#35330);
#28435=AXIS2_PLACEMENT_3D('',#65884,#35332,#35333);
#28436=AXIS2_PLACEMENT_3D('',#65886,#35335,#35336);
#28437=AXIS2_PLACEMENT_3D('',#65888,#35338,#35339);
#28438=AXIS2_PLACEMENT_3D('',#65890,#35341,#35342);
#28439=AXIS2_PLACEMENT_3D('',#65891,#35343,#35344);
#28440=AXIS2_PLACEMENT_3D('',#65897,#35348,#35349);
#28441=AXIS2_PLACEMENT_3D('',#65900,#35351,#35352);
#28442=AXIS2_PLACEMENT_3D('',#65901,#35353,#35354);
#28443=AXIS2_PLACEMENT_3D('',#65904,#35356,#35357);
#28444=AXIS2_PLACEMENT_3D('',#65905,#35358,#35359);
#28445=AXIS2_PLACEMENT_3D('',#65909,#35362,#35363);
#28446=AXIS2_PLACEMENT_3D('',#65911,#35364,#35365);
#28447=AXIS2_PLACEMENT_3D('',#65913,#35367,#35368);
#28448=AXIS2_PLACEMENT_3D('',#65914,#35369,#35370);
#28449=AXIS2_PLACEMENT_3D('',#65915,#35371,#35372);
#28450=AXIS2_PLACEMENT_3D('',#65916,#35373,#35374);
#28451=AXIS2_PLACEMENT_3D('',#65920,#35376,#35377);
#28452=AXIS2_PLACEMENT_3D('',#65922,#35379,#35380);
#28453=AXIS2_PLACEMENT_3D('',#65926,#35383,#35384);
#28454=AXIS2_PLACEMENT_3D('',#65929,#35386,#35387);
#28455=AXIS2_PLACEMENT_3D('',#65930,#35388,#35389);
#28456=AXIS2_PLACEMENT_3D('',#65949,#35391,#35392);
#28457=AXIS2_PLACEMENT_3D('',#65953,#35395,#35396);
#28458=AXIS2_PLACEMENT_3D('',#65957,#35398,#35399);
#28459=AXIS2_PLACEMENT_3D('',#65959,#35401,#35402);
#28460=AXIS2_PLACEMENT_3D('',#65963,#35405,#35406);
#28461=AXIS2_PLACEMENT_3D('',#65966,#35408,#35409);
#28462=AXIS2_PLACEMENT_3D('',#65967,#35410,#35411);
#28463=AXIS2_PLACEMENT_3D('',#65971,#35414,#35415);
#28464=AXIS2_PLACEMENT_3D('',#65974,#35417,#35418);
#28465=AXIS2_PLACEMENT_3D('',#65975,#35419,#35420);
#28466=AXIS2_PLACEMENT_3D('',#65977,#35422,#35423);
#28467=AXIS2_PLACEMENT_3D('',#65998,#35425,#35426);
#28468=AXIS2_PLACEMENT_3D('',#66000,#35428,#35429);
#34889=DIRECTION('axis',(0.,0.,1.));
#34890=DIRECTION('refdir',(1.,0.,0.));
#34891=DIRECTION('center_axis',(-1.,0.,0.));
#34892=DIRECTION('ref_axis',(0.,0.,1.));
#34893=DIRECTION('',(0.,0.707106781186548,-0.707106781186548));
#34894=DIRECTION('center_axis',(-1.,0.,0.));
#34895=DIRECTION('ref_axis',(0.,0.,1.));
#34896=DIRECTION('',(0.,0.707106781186547,-0.707106781186547));
#34897=DIRECTION('center_axis',(1.,0.,0.));
#34898=DIRECTION('ref_axis',(0.,0.,1.));
#34899=DIRECTION('center_axis',(1.,0.,0.));
#34900=DIRECTION('ref_axis',(0.,-0.707106781186548,-0.707106781186547));
#34901=DIRECTION('center_axis',(-1.,0.,0.));
#34902=DIRECTION('ref_axis',(0.,0.,1.));
#34903=DIRECTION('',(-0.707104308763577,0.500001748260936,-0.500001748260935));
#34904=DIRECTION('',(0.707104308763577,0.500001748260935,-0.500001748260936));
#34905=DIRECTION('center_axis',(1.,0.,0.));
#34906=DIRECTION('ref_axis',(0.,1.,0.));
#34907=DIRECTION('center_axis',(-1.,0.,0.));
#34908=DIRECTION('ref_axis',(0.,-0.707106781186547,-0.707106781186548));
#34909=DIRECTION('center_axis',(-1.,0.,0.));
#34910=DIRECTION('ref_axis',(0.,0.,1.));
#34911=DIRECTION('center_axis',(-1.,0.,0.));
#34912=DIRECTION('ref_axis',(0.,0.707106781186548,-0.707106781186547));
#34913=DIRECTION('center_axis',(-1.,0.,0.));
#34914=DIRECTION('ref_axis',(0.,0.,-1.));
#34915=DIRECTION('center_axis',(1.,0.,0.));
#34916=DIRECTION('ref_axis',(0.,1.,0.));
#34917=DIRECTION('center_axis',(-1.,0.,0.));
#34918=DIRECTION('ref_axis',(0.,0.707106781186548,-0.707106781186547));
#34919=DIRECTION('center_axis',(-1.,0.,0.));
#34920=DIRECTION('ref_axis',(0.,0.,1.));
#34921=DIRECTION('center_axis',(-1.,0.,0.));
#34922=DIRECTION('ref_axis',(0.,0.707106781186547,0.707106781186548));
#34923=DIRECTION('center_axis',(-1.,0.,0.));
#34924=DIRECTION('ref_axis',(0.,0.,-1.));
#34925=DIRECTION('center_axis',(1.,0.,0.));
#34926=DIRECTION('ref_axis',(0.,0.,-1.));
#34927=DIRECTION('center_axis',(-1.,0.,0.));
#34928=DIRECTION('ref_axis',(0.,0.,-1.));
#34929=DIRECTION('',(1.,0.,0.));
#34930=DIRECTION('',(-1.,0.,0.));
#34931=DIRECTION('center_axis',(1.,0.,0.));
#34932=DIRECTION('ref_axis',(0.,0.,-1.));
#34933=DIRECTION('',(1.,0.,0.));
#34934=DIRECTION('',(-1.,0.,0.));
#34935=DIRECTION('center_axis',(-1.,0.,0.));
#34936=DIRECTION('ref_axis',(0.,0.,-1.));
#34937=DIRECTION('center_axis',(1.,0.,0.));
#34938=DIRECTION('ref_axis',(0.,-0.870991239054279,-0.491298546192324));
#34939=DIRECTION('',(1.,0.,0.));
#34940=DIRECTION('center_axis',(-1.,0.,0.));
#34941=DIRECTION('ref_axis',(0.,0.707106781186547,0.707106781186548));
#34942=DIRECTION('center_axis',(1.,0.,0.));
#34943=DIRECTION('ref_axis',(0.,-0.491298546192324,0.870991239054279));
#34944=DIRECTION('',(1.,0.,0.));
#34945=DIRECTION('center_axis',(-1.,0.,0.));
#34946=DIRECTION('ref_axis',(0.,0.707106781186548,-0.707106781186547));
#34947=DIRECTION('center_axis',(1.,0.,0.));
#34948=DIRECTION('ref_axis',(0.,0.707106781186548,-0.707106781186547));
#34949=DIRECTION('center_axis',(-1.,0.,0.));
#34950=DIRECTION('ref_axis',(0.,0.707106781186548,-0.707106781186547));
#34951=DIRECTION('',(-1.,0.,0.));
#34952=DIRECTION('center_axis',(1.,0.,0.));
#34953=DIRECTION('ref_axis',(0.,-0.707106781186547,-0.707106781186548));
#34954=DIRECTION('center_axis',(-1.,0.,0.));
#34955=DIRECTION('ref_axis',(0.,-0.707106781186547,-0.707106781186548));
#34956=DIRECTION('',(-1.,0.,0.));
#34957=DIRECTION('center_axis',(-1.,0.,0.));
#34958=DIRECTION('ref_axis',(0.,-0.707106781186547,-0.707106781186548));
#34959=DIRECTION('center_axis',(-1.,0.,0.));
#34960=DIRECTION('ref_axis',(0.,0.,1.));
#34961=DIRECTION('center_axis',(-1.,0.,0.));
#34962=DIRECTION('ref_axis',(0.,0.,1.));
#34963=DIRECTION('',(-1.,0.,0.));
#34964=DIRECTION('',(1.,0.,0.));
#34965=DIRECTION('center_axis',(-1.,0.,0.));
#34966=DIRECTION('ref_axis',(0.,0.,1.));
#34967=DIRECTION('',(1.,0.,0.));
#34968=DIRECTION('center_axis',(-1.,0.,0.));
#34969=DIRECTION('ref_axis',(0.,-0.707106781186547,-0.707106781186548));
#34970=DIRECTION('',(1.,0.,0.));
#34971=DIRECTION('center_axis',(-1.,0.,0.));
#34972=DIRECTION('ref_axis',(0.,0.,1.));
#34973=DIRECTION('',(-1.,0.,0.));
#34974=DIRECTION('center_axis',(-1.,0.,0.));
#34975=DIRECTION('ref_axis',(0.,0.,1.));
#34976=DIRECTION('',(0.,-0.707106781186547,0.707106781186547));
#34977=DIRECTION('',(0.,-0.707106781186547,0.707106781186547));
#34978=DIRECTION('center_axis',(0.,0.707106781186549,0.707106781186546));
#34979=DIRECTION('ref_axis',(-1.,0.,0.));
#34980=DIRECTION('',(0.,0.707106781186549,0.707106781186546));
#34981=DIRECTION('center_axis',(0.,0.707106781186548,0.707106781186548));
#34982=DIRECTION('ref_axis',(-1.,0.,0.));
#34983=DIRECTION('center_axis',(0.,0.707106781186549,0.707106781186546));
#34984=DIRECTION('ref_axis',(1.,0.,0.));
#34985=DIRECTION('center_axis',(0.,-0.707106781186549,-0.707106781186546));
#34986=DIRECTION('ref_axis',(-1.,0.,0.));
#34987=DIRECTION('center_axis',(0.,-0.707106781186549,-0.707106781186546));
#34988=DIRECTION('ref_axis',(-1.,0.,0.));
#34989=DIRECTION('center_axis',(0.,-0.707106781186549,-0.707106781186546));
#34990=DIRECTION('ref_axis',(-1.,0.,0.));
#34991=DIRECTION('center_axis',(0.,-0.707106781186549,-0.707106781186546));
#34992=DIRECTION('ref_axis',(-1.,0.,0.));
#34993=DIRECTION('',(0.,-0.707106781186549,-0.707106781186546));
#34994=DIRECTION('center_axis',(0.,0.707106781186549,0.707106781186546));
#34995=DIRECTION('ref_axis',(1.,0.,0.));
#34996=DIRECTION('center_axis',(0.,-0.707106781186549,-0.707106781186546));
#34997=DIRECTION('ref_axis',(-1.,0.,0.));
#34998=DIRECTION('center_axis',(0.,-0.707106781186549,-0.707106781186546));
#34999=DIRECTION('ref_axis',(-1.,0.,0.));
#35000=DIRECTION('center_axis',(0.,0.707106781186548,0.707106781186548));
#35001=DIRECTION('ref_axis',(-1.,0.,0.));
#35002=DIRECTION('',(0.,-0.707106781186549,-0.707106781186546));
#35003=DIRECTION('center_axis',(0.,0.707106781186548,0.707106781186548));
#35004=DIRECTION('ref_axis',(1.,0.,0.));
#35005=DIRECTION('center_axis',(0.,0.707106781186548,0.707106781186548));
#35006=DIRECTION('ref_axis',(1.,0.,0.));
#35007=DIRECTION('center_axis',(0.,-0.707106781186549,-0.707106781186546));
#35008=DIRECTION('ref_axis',(-5.0532154980743E-16,0.707106781186546,-0.707106781186549));
#35009=DIRECTION('center_axis',(0.,0.707106781186549,0.707106781186546));
#35010=DIRECTION('ref_axis',(-5.0532154980743E-16,-0.707106781186546,0.707106781186549));
#35011=DIRECTION('center_axis',(0.,0.707106781186549,0.707106781186546));
#35012=DIRECTION('ref_axis',(-1.,0.,0.));
#35013=DIRECTION('center_axis',(0.,-0.707106781186548,-0.707106781186548));
#35014=DIRECTION('ref_axis',(0.,-0.707106781186548,0.707106781186548));
#35015=DIRECTION('',(0.707104308763575,-0.500001748260937,0.500001748260937));
#35016=DIRECTION('',(0.,-0.707106781186547,0.707106781186547));
#35017=DIRECTION('',(-1.,0.,0.));
#35018=DIRECTION('',(0.,0.707106781186547,-0.707106781186547));
#35019=DIRECTION('',(1.,0.,0.));
#35020=DIRECTION('center_axis',(0.,-0.707106781186548,-0.707106781186548));
#35021=DIRECTION('ref_axis',(-1.,0.,0.));
#35022=DIRECTION('center_axis',(0.,-0.707106781186549,-0.707106781186546));
#35023=DIRECTION('ref_axis',(-1.,0.,0.));
#35024=DIRECTION('',(0.,-0.707106781186549,-0.707106781186546));
#35025=DIRECTION('center_axis',(0.,0.707106781186549,0.707106781186546));
#35026=DIRECTION('ref_axis',(-1.,0.,0.));
#35027=DIRECTION('center_axis',(0.,-0.707106781186548,-0.707106781186548));
#35028=DIRECTION('ref_axis',(-1.,0.,0.));
#35029=DIRECTION('',(0.,0.707106781186549,0.707106781186546));
#35030=DIRECTION('center_axis',(0.,0.707106781186549,0.707106781186546));
#35031=DIRECTION('ref_axis',(-1.,0.,0.));
#35032=DIRECTION('center_axis',(0.,-0.707106781186549,-0.707106781186546));
#35033=DIRECTION('ref_axis',(0.,0.707106781186546,-0.707106781186549));
#35034=DIRECTION('center_axis',(0.,0.707106781186549,0.707106781186546));
#35035=DIRECTION('ref_axis',(-1.,0.,0.));
#35036=DIRECTION('center_axis',(0.,0.707106781186549,0.707106781186546));
#35037=DIRECTION('ref_axis',(-1.,0.,0.));
#35038=DIRECTION('',(0.,0.707106781186549,0.707106781186546));
#35039=DIRECTION('center_axis',(0.,0.707106781186549,0.707106781186546));
#35040=DIRECTION('ref_axis',(-1.,0.,0.));
#35041=DIRECTION('center_axis',(0.,-0.707106781186549,-0.707106781186546));
#35042=DIRECTION('ref_axis',(0.,0.707106781186546,-0.707106781186549));
#35043=DIRECTION('',(1.,0.,0.));
#35044=DIRECTION('center_axis',(0.,-0.707106781186548,-0.707106781186548));
#35045=DIRECTION('ref_axis',(0.,-0.707106781186548,0.707106781186548));
#35046=DIRECTION('',(-0.707104308763575,-0.500001748260937,0.500001748260937));
#35047=DIRECTION('',(-1.,0.,0.));
#35048=DIRECTION('',(0.,0.707106781186547,-0.707106781186547));
#35049=DIRECTION('',(1.,0.,0.));
#35050=DIRECTION('',(0.,-0.707106781186547,0.707106781186547));
#35051=DIRECTION('center_axis',(-1.,0.,0.));
#35052=DIRECTION('ref_axis',(0.,0.,1.));
#35053=DIRECTION('center_axis',(1.,0.,0.));
#35054=DIRECTION('ref_axis',(0.,0.,1.));
#35055=DIRECTION('',(0.,0.707106781186547,0.707106781186547));
#35056=DIRECTION('',(0.,-0.707106781186547,0.707106781186547));
#35057=DIRECTION('',(0.,-0.707106781186547,-0.707106781186547));
#35058=DIRECTION('center_axis',(1.,0.,0.));
#35059=DIRECTION('ref_axis',(0.,0.,1.));
#35060=DIRECTION('center_axis',(-1.,0.,0.));
#35061=DIRECTION('ref_axis',(0.,0.,1.));
#35062=DIRECTION('center_axis',(1.,0.,0.));
#35063=DIRECTION('ref_axis',(0.,0.,1.));
#35064=DIRECTION('center_axis',(-1.,0.,0.));
#35065=DIRECTION('ref_axis',(0.,0.,1.));
#35066=DIRECTION('center_axis',(-1.,0.,0.));
#35067=DIRECTION('ref_axis',(0.,0.,1.));
#35068=DIRECTION('center_axis',(-1.,0.,0.));
#35069=DIRECTION('ref_axis',(0.,0.,1.));
#35070=DIRECTION('center_axis',(-1.,0.,0.));
#35071=DIRECTION('ref_axis',(0.,0.707106781186547,0.707106781186548));
#35072=DIRECTION('center_axis',(-1.,0.,0.));
#35073=DIRECTION('ref_axis',(0.,0.,-1.));
#35074=DIRECTION('center_axis',(-1.,0.,0.));
#35075=DIRECTION('ref_axis',(0.,-0.707106781186548,0.707106781186547));
#35076=DIRECTION('center_axis',(-1.,0.,0.));
#35077=DIRECTION('ref_axis',(0.,0.,1.));
#35078=DIRECTION('center_axis',(-1.,0.,0.));
#35079=DIRECTION('ref_axis',(0.,-0.707106781186548,0.707106781186547));
#35080=DIRECTION('center_axis',(-1.,0.,0.));
#35081=DIRECTION('ref_axis',(0.,0.,-1.));
#35082=DIRECTION('center_axis',(-1.,0.,0.));
#35083=DIRECTION('ref_axis',(0.,-0.707106781186547,-0.707106781186548));
#35084=DIRECTION('center_axis',(-1.,0.,0.));
#35085=DIRECTION('ref_axis',(0.,0.,1.));
#35086=DIRECTION('center_axis',(-1.,0.,0.));
#35087=DIRECTION('ref_axis',(0.,0.,1.));
#35088=DIRECTION('',(0.,0.707106781186547,0.707106781186547));
#35089=DIRECTION('',(0.,0.707106781186547,-0.707106781186547));
#35090=DIRECTION('',(0.,-0.707106781186547,-0.707106781186547));
#35091=DIRECTION('center_axis',(-1.,0.,0.));
#35092=DIRECTION('ref_axis',(0.,0.,1.));
#35093=DIRECTION('center_axis',(-1.,0.,0.));
#35094=DIRECTION('ref_axis',(0.,0.,1.));
#35095=DIRECTION('',(-1.,0.,0.));
#35096=DIRECTION('center_axis',(-1.,0.,0.));
#35097=DIRECTION('ref_axis',(0.,0.,1.));
#35098=DIRECTION('',(1.,0.,0.));
#35099=DIRECTION('center_axis',(-1.,0.,0.));
#35100=DIRECTION('ref_axis',(0.,0.,1.));
#35101=DIRECTION('',(-1.,0.,0.));
#35102=DIRECTION('',(1.,0.,0.));
#35103=DIRECTION('center_axis',(-1.,0.,0.));
#35104=DIRECTION('ref_axis',(0.,0.,1.));
#35105=DIRECTION('center_axis',(0.,0.707106781186548,0.707106781186548));
#35106=DIRECTION('ref_axis',(1.,0.,0.));
#35107=DIRECTION('center_axis',(0.,-0.707106781186548,-0.707106781186548));
#35108=DIRECTION('ref_axis',(1.,0.,0.));
#35109=DIRECTION('',(0.,0.707106781186548,0.707106781186548));
#35110=DIRECTION('center_axis',(0.,-0.707106781186548,0.707106781186548));
#35111=DIRECTION('ref_axis',(-1.,0.,0.));
#35112=DIRECTION('',(-1.,0.,0.));
#35113=DIRECTION('center_axis',(0.,0.707106781186548,-0.707106781186548));
#35114=DIRECTION('ref_axis',(-1.,0.,0.));
#35115=DIRECTION('',(1.,0.,0.));
#35116=DIRECTION('center_axis',(0.,0.707106781186548,0.707106781186548));
#35117=DIRECTION('ref_axis',(1.,0.,0.));
#35118=DIRECTION('center_axis',(1.,0.,0.));
#35119=DIRECTION('ref_axis',(0.,0.870991239054279,0.491298546192324));
#35120=DIRECTION('center_axis',(-1.,0.,0.));
#35121=DIRECTION('ref_axis',(0.,-0.707106781186547,-0.707106781186548));
#35122=DIRECTION('',(1.,0.,0.));
#35123=DIRECTION('',(-1.,0.,0.));
#35124=DIRECTION('center_axis',(1.,0.,0.));
#35125=DIRECTION('ref_axis',(0.,0.491298546192324,-0.870991239054279));
#35126=DIRECTION('center_axis',(-1.,0.,0.));
#35127=DIRECTION('ref_axis',(0.,-0.707106781186548,0.707106781186547));
#35128=DIRECTION('',(1.,0.,0.));
#35129=DIRECTION('',(-1.,0.,0.));
#35130=DIRECTION('center_axis',(1.,0.,0.));
#35131=DIRECTION('ref_axis',(0.,0.707106781186547,0.707106781186548));
#35132=DIRECTION('',(-1.,0.,0.));
#35133=DIRECTION('center_axis',(-1.,0.,0.));
#35134=DIRECTION('ref_axis',(0.,0.707106781186547,0.707106781186548));
#35135=DIRECTION('',(1.,0.,0.));
#35136=DIRECTION('center_axis',(1.,0.,0.));
#35137=DIRECTION('ref_axis',(0.,1.22464679914735E-16,1.));
#35138=DIRECTION('center_axis',(-1.,0.,0.));
#35139=DIRECTION('ref_axis',(0.,0.,-1.));
#35140=DIRECTION('',(1.,0.,0.));
#35141=DIRECTION('center_axis',(1.,0.,0.));
#35142=DIRECTION('ref_axis',(0.,0.,-1.));
#35143=DIRECTION('center_axis',(-1.,0.,0.));
#35144=DIRECTION('ref_axis',(0.,0.,-1.));
#35145=DIRECTION('center_axis',(1.,0.,0.));
#35146=DIRECTION('ref_axis',(0.,-0.707106781186548,0.707106781186547));
#35147=DIRECTION('',(-1.,0.,0.));
#35148=DIRECTION('center_axis',(-1.,0.,0.));
#35149=DIRECTION('ref_axis',(0.,-0.707106781186548,0.707106781186547));
#35150=DIRECTION('center_axis',(1.,0.,0.));
#35151=DIRECTION('ref_axis',(0.,1.,0.));
#35152=DIRECTION('center_axis',(-1.,0.,0.));
#35153=DIRECTION('ref_axis',(0.,0.,1.));
#35154=DIRECTION('center_axis',(1.,0.,0.));
#35155=DIRECTION('ref_axis',(0.,1.,0.));
#35156=DIRECTION('center_axis',(-1.,0.,0.));
#35157=DIRECTION('ref_axis',(0.,0.,1.));
#35158=DIRECTION('center_axis',(-1.,0.,0.));
#35159=DIRECTION('ref_axis',(0.,0.,1.));
#35160=DIRECTION('center_axis',(-0.946028810149193,-0.324082536351007,-1.06892949644448E-9));
#35161=DIRECTION('ref_axis',(-0.0238519321544925,0.069626133465603,0.997287965871005));
#35162=DIRECTION('',(1.,0.,0.));
#35163=DIRECTION('center_axis',(0.946028810160761,0.324082536317239,-1.73103110021756E-13));
#35164=DIRECTION('ref_axis',(-0.00756181520538782,0.0220736825960291,0.999727748683335));
#35165=DIRECTION('',(1.,0.,0.));
#35166=DIRECTION('center_axis',(-1.,0.,0.));
#35167=DIRECTION('ref_axis',(0.,0.,1.));
#35168=DIRECTION('',(1.,0.,0.));
#35169=DIRECTION('center_axis',(1.,0.,0.));
#35170=DIRECTION('ref_axis',(0.,0.,1.));
#35171=DIRECTION('',(-1.,0.,0.));
#35172=DIRECTION('center_axis',(-1.,0.,0.));
#35173=DIRECTION('ref_axis',(0.,0.,1.));
#35174=DIRECTION('',(1.,0.,0.));
#35175=DIRECTION('center_axis',(1.,0.,0.));
#35176=DIRECTION('ref_axis',(0.,0.,1.));
#35177=DIRECTION('',(1.,0.,0.));
#35178=DIRECTION('center_axis',(1.,0.,0.));
#35179=DIRECTION('ref_axis',(0.,0.,1.));
#35180=DIRECTION('',(-1.,0.,0.));
#35181=DIRECTION('center_axis',(-1.,0.,0.));
#35182=DIRECTION('ref_axis',(0.,0.,1.));
#35183=DIRECTION('',(1.,0.,0.));
#35184=DIRECTION('',(-1.,0.,0.));
#35185=DIRECTION('center_axis',(-0.500000000011387,-0.866025403777865,-1.13502270606945E-13));
#35186=DIRECTION('ref_axis',(0.866025403777865,-0.500000000011387,-1.2232312709768E-10));
#35187=DIRECTION('center_axis',(0.500000000011405,-0.866025403777854,2.15654314153191E-13));
#35188=DIRECTION('ref_axis',(0.866025403777854,0.500000000011405,7.56457705137375E-10));
#35189=DIRECTION('',(-1.,0.,0.));
#35190=DIRECTION('center_axis',(-0.500000000001134,0.866025403783784,1.17302365318434E-14));
#35191=DIRECTION('ref_axis',(0.866025403783784,0.500000000001134,-3.36774821015014E-10));
#35192=DIRECTION('center_axis',(0.500000000001136,0.866025403783783,-1.95503942197372E-14));
#35193=DIRECTION('ref_axis',(0.866025403783783,-0.500000000001136,1.13706776558401E-10));
#35194=DIRECTION('center_axis',(0.855183382509445,0.518325556267202,0.));
#35195=DIRECTION('ref_axis',(-0.518325556267202,0.855183382509445,0.));
#35196=DIRECTION('',(1.,0.,0.));
#35197=DIRECTION('center_axis',(0.855183382508505,0.518325556268753,-1.92327333756619E-13));
#35198=DIRECTION('ref_axis',(-0.00559375624087415,0.00922911734785472,0.999941764946388));
#35199=DIRECTION('center_axis',(-1.,0.,0.));
#35200=DIRECTION('ref_axis',(0.,0.,1.));
#35201=DIRECTION('',(1.,0.,0.));
#35202=DIRECTION('center_axis',(1.,0.,0.));
#35203=DIRECTION('ref_axis',(0.,0.,1.));
#35204=DIRECTION('',(-1.,0.,0.));
#35205=DIRECTION('center_axis',(-1.,0.,0.));
#35206=DIRECTION('ref_axis',(0.,0.,1.));
#35207=DIRECTION('center_axis',(0.829037572548643,-0.559192903480234,-1.64064661511221E-13));
#35208=DIRECTION('ref_axis',(-0.0360858435021883,-0.0534994630911657,0.997915637390102));
#35209=DIRECTION('',(-1.,0.,0.));
#35210=DIRECTION('center_axis',(-0.82903757255312,0.559192903473596,0.));
#35211=DIRECTION('ref_axis',(0.559192903473596,0.82903757255312,0.));
#35212=DIRECTION('center_axis',(-0.500000000011404,0.866025403777855,1.81603632971102E-13));
#35213=DIRECTION('ref_axis',(0.866025403777855,0.500000000011404,-1.23583351950854E-10));
#35214=DIRECTION('',(1.,0.,0.));
#35215=DIRECTION('center_axis',(0.500000000001135,-0.866025403783783,-7.82015768789461E-15));
#35216=DIRECTION('ref_axis',(0.866025403783783,0.500000000001135,1.8743640553155E-10));
#35217=DIRECTION('center_axis',(-0.500000000001136,-0.866025403783783,-1.56403153757889E-14));
#35218=DIRECTION('ref_axis',(0.866025403783783,-0.500000000001136,-1.67428462619296E-10));
#35219=DIRECTION('',(1.,0.,0.));
#35220=DIRECTION('center_axis',(0.500000000011388,0.866025403777864,-9.08018164855533E-14));
#35221=DIRECTION('ref_axis',(0.866025403777864,-0.500000000011388,8.55286471205808E-10));
#35222=DIRECTION('center_axis',(-1.,0.,0.));
#35223=DIRECTION('ref_axis',(0.,0.,1.));
#35224=DIRECTION('center_axis',(1.,0.,0.));
#35225=DIRECTION('ref_axis',(0.,0.,1.));
#35226=DIRECTION('',(-1.,0.,0.));
#35227=DIRECTION('center_axis',(1.,0.,0.));
#35228=DIRECTION('ref_axis',(0.,0.,1.));
#35229=DIRECTION('',(1.,0.,0.));
#35230=DIRECTION('center_axis',(-1.,0.,0.));
#35231=DIRECTION('ref_axis',(0.,0.,1.));
#35232=DIRECTION('',(-1.,0.,0.));
#35233=DIRECTION('center_axis',(-1.,0.,0.));
#35234=DIRECTION('ref_axis',(0.,0.,1.));
#35235=DIRECTION('',(-1.,0.,0.));
#35236=DIRECTION('center_axis',(1.,0.,0.));
#35237=DIRECTION('ref_axis',(0.,1.,0.));
#35238=DIRECTION('',(0.,0.,1.));
#35239=DIRECTION('',(0.,0.,1.));
#35240=DIRECTION('center_axis',(0.,1.,0.));
#35241=DIRECTION('ref_axis',(1.,0.,0.));
#35242=DIRECTION('',(0.,0.,1.));
#35243=DIRECTION('center_axis',(0.,1.,0.));
#35244=DIRECTION('ref_axis',(1.,0.,0.));
#35245=DIRECTION('',(0.,0.,1.));
#35246=DIRECTION('center_axis',(1.,0.,0.));
#35247=DIRECTION('ref_axis',(0.,1.,0.));
#35248=DIRECTION('',(0.,0.,1.));
#35249=DIRECTION('center_axis',(0.,-1.,0.));
#35250=DIRECTION('ref_axis',(0.,0.,-1.));
#35251=DIRECTION('',(0.,0.,1.));
#35252=DIRECTION('center_axis',(-1.,0.,0.));
#35253=DIRECTION('ref_axis',(0.,0.,1.));
#35254=DIRECTION('',(0.,0.,1.));
#35255=DIRECTION('center_axis',(0.,1.,0.));
#35256=DIRECTION('ref_axis',(1.,0.,0.));
#35257=DIRECTION('',(0.,0.,1.));
#35258=DIRECTION('center_axis',(-1.,0.,0.));
#35259=DIRECTION('ref_axis',(0.,0.,1.));
#35260=DIRECTION('center_axis',(0.855183382508501,0.518325556268759,0.));
#35261=DIRECTION('ref_axis',(0.,0.,-1.));
#35262=DIRECTION('',(0.,0.,1.));
#35263=DIRECTION('center_axis',(-0.855183382508501,-0.518325556268759,0.));
#35264=DIRECTION('ref_axis',(-0.518325556268759,0.855183382508501,0.));
#35265=DIRECTION('',(0.,0.,1.));
#35266=DIRECTION('center_axis',(0.,1.,0.));
#35267=DIRECTION('ref_axis',(1.,0.,0.));
#35268=DIRECTION('',(0.,0.,1.));
#35269=DIRECTION('',(-1.,0.,0.));
#35270=DIRECTION('center_axis',(-0.855183382509445,-0.518325556267202,0.));
#35271=DIRECTION('ref_axis',(-0.518325556267202,0.855183382509445,0.));
#35272=DIRECTION('',(0.,0.,1.));
#35273=DIRECTION('center_axis',(-0.855183382509445,-0.518325556267202,0.));
#35274=DIRECTION('ref_axis',(-0.518325556267202,0.855183382509445,0.));
#35275=DIRECTION('center_axis',(0.,-1.,0.));
#35276=DIRECTION('ref_axis',(0.,0.,-1.));
#35277=DIRECTION('',(0.,0.,1.));
#35278=DIRECTION('',(1.,0.,0.));
#35279=DIRECTION('',(0.,0.,1.));
#35280=DIRECTION('center_axis',(0.829037572548639,-0.55919290348024,0.));
#35281=DIRECTION('ref_axis',(0.,0.,-1.));
#35282=DIRECTION('',(0.,0.,1.));
#35283=DIRECTION('center_axis',(-0.829037572548647,0.559192903480227,3.27863405626968E-13));
#35284=DIRECTION('ref_axis',(-0.0128476572568338,-0.0190474351859132,0.999736031618271));
#35285=DIRECTION('center_axis',(-1.,0.,0.));
#35286=DIRECTION('ref_axis',(0.,0.,1.));
#35287=DIRECTION('',(0.,0.,1.));
#35288=DIRECTION('center_axis',(1.,0.,0.));
#35289=DIRECTION('ref_axis',(0.,0.,1.));
#35290=DIRECTION('center_axis',(0.,-1.,0.));
#35291=DIRECTION('ref_axis',(0.,0.,-1.));
#35292=DIRECTION('',(0.,0.,1.));
#35293=DIRECTION('',(1.,0.,0.));
#35294=DIRECTION('center_axis',(1.,0.,0.));
#35295=DIRECTION('ref_axis',(0.,1.,0.));
#35296=DIRECTION('',(0.,0.,1.));
#35297=DIRECTION('center_axis',(-1.,0.,0.));
#35298=DIRECTION('ref_axis',(0.,0.,1.));
#35299=DIRECTION('center_axis',(0.,1.,0.));
#35300=DIRECTION('ref_axis',(1.,0.,0.));
#35301=DIRECTION('',(0.,0.,1.));
#35302=DIRECTION('',(-1.,0.,0.));
#35303=DIRECTION('center_axis',(-1.,0.,0.));
#35304=DIRECTION('ref_axis',(0.,0.,1.));
#35305=DIRECTION('center_axis',(1.,0.,0.));
#35306=DIRECTION('ref_axis',(0.,0.,1.));
#35307=DIRECTION('center_axis',(-0.82903757255312,0.559192903473596,0.));
#35308=DIRECTION('ref_axis',(0.,0.,1.));
#35309=DIRECTION('center_axis',(0.82903757255312,-0.559192903473596,0.));
#35310=DIRECTION('ref_axis',(0.559192903473596,0.82903757255312,0.));
#35311=DIRECTION('center_axis',(-1.,0.,0.));
#35312=DIRECTION('ref_axis',(0.,0.,1.));
#35313=DIRECTION('center_axis',(-1.,0.,0.));
#35314=DIRECTION('ref_axis',(0.,0.,1.));
#35315=DIRECTION('center_axis',(0.500000000001141,-0.86602540378378,9.20240256887291E-14));
#35316=DIRECTION('ref_axis',(0.86602540378378,0.500000000001141,4.288515013244E-11));
#35317=DIRECTION('',(1.,0.,0.));
#35318=DIRECTION('center_axis',(-0.500000000011408,0.866025403777852,-2.56081897120736E-13));
#35319=DIRECTION('ref_axis',(0.866025403777852,0.500000000011408,4.05069188609369E-10));
#35320=DIRECTION('center_axis',(0.500000000011408,0.866025403777853,-2.33813906066936E-13));
#35321=DIRECTION('ref_axis',(0.866025403777853,-0.500000000011407,3.46137901213225E-10));
#35322=DIRECTION('',(1.,0.,0.));
#35323=DIRECTION('center_axis',(-0.50000000000114,-0.86602540378378,7.66866880739418E-14));
#35324=DIRECTION('ref_axis',(0.86602540378378,-0.50000000000114,2.49921069793427E-11));
#35325=DIRECTION('center_axis',(0.500000000011394,-0.866025403777861,0.));
#35326=DIRECTION('ref_axis',(0.,0.,-1.));
#35327=DIRECTION('',(0.,0.,1.));
#35328=DIRECTION('',(0.,0.,1.));
#35329=DIRECTION('center_axis',(-0.500000000011394,-0.866025403777861,0.));
#35330=DIRECTION('ref_axis',(-0.866025403777861,0.500000000011394,0.));
#35331=DIRECTION('',(0.,0.,1.));
#35332=DIRECTION('center_axis',(0.,-1.,0.));
#35333=DIRECTION('ref_axis',(0.,0.,-1.));
#35334=DIRECTION('',(0.,0.,1.));
#35335=DIRECTION('center_axis',(-0.500000000001135,0.866025403783784,0.));
#35336=DIRECTION('ref_axis',(0.,0.,1.));
#35337=DIRECTION('',(0.,0.,1.));
#35338=DIRECTION('center_axis',(0.500000000001135,0.866025403783784,0.));
#35339=DIRECTION('ref_axis',(0.,0.,-1.));
#35340=DIRECTION('',(0.,0.,1.));
#35341=DIRECTION('center_axis',(0.,-1.,0.));
#35342=DIRECTION('ref_axis',(0.,0.,-1.));
#35343=DIRECTION('center_axis',(0.,1.,0.));
#35344=DIRECTION('ref_axis',(1.,0.,0.));
#35345=DIRECTION('',(0.,0.,1.));
#35346=DIRECTION('',(-1.,0.,0.));
#35347=DIRECTION('',(0.,0.,1.));
#35348=DIRECTION('center_axis',(-0.500000000001135,-0.866025403783784,0.));
#35349=DIRECTION('ref_axis',(-0.866025403783784,0.500000000001135,0.));
#35350=DIRECTION('',(0.,0.,1.));
#35351=DIRECTION('center_axis',(0.500000000001142,0.866025403783779,1.0736136330352E-13));
#35352=DIRECTION('ref_axis',(0.866025403783779,-0.500000000001142,-1.03942187968842E-11));
#35353=DIRECTION('center_axis',(0.500000000001135,-0.866025403783784,0.));
#35354=DIRECTION('ref_axis',(0.,0.,-1.));
#35355=DIRECTION('',(0.,0.,1.));
#35356=DIRECTION('center_axis',(-0.500000000001139,0.866025403783781,6.13493504591534E-14));
#35357=DIRECTION('ref_axis',(0.866025403783781,0.500000000001139,4.35266584402982E-13));
#35358=DIRECTION('center_axis',(0.,1.,0.));
#35359=DIRECTION('ref_axis',(1.,0.,0.));
#35360=DIRECTION('',(0.,0.,1.));
#35361=DIRECTION('',(-1.,0.,0.));
#35362=DIRECTION('center_axis',(0.500000000011394,0.866025403777861,0.));
#35363=DIRECTION('ref_axis',(0.,0.,-1.));
#35364=DIRECTION('center_axis',(-0.50000000001141,-0.866025403777851,-2.89483883701782E-13));
#35365=DIRECTION('ref_axis',(0.866025403777851,-0.50000000001141,-1.20134541954323E-10));
#35366=DIRECTION('',(0.,0.,1.));
#35367=DIRECTION('center_axis',(-0.500000000011394,0.866025403777861,0.));
#35368=DIRECTION('ref_axis',(0.,0.,1.));
#35369=DIRECTION('center_axis',(0.500000000011409,-0.866025403777852,-2.67215892647728E-13));
#35370=DIRECTION('ref_axis',(0.866025403777852,0.500000000011409,1.29145984166572E-9));
#35371=DIRECTION('center_axis',(-1.,0.,0.));
#35372=DIRECTION('ref_axis',(0.,0.,1.));
#35373=DIRECTION('center_axis',(0.946028810160758,0.324082536317247,0.));
#35374=DIRECTION('ref_axis',(0.,0.,-1.));
#35375=DIRECTION('',(0.,0.,1.));
#35376=DIRECTION('center_axis',(-0.94602881016076,-0.324082536317244,6.79718201582214E-14));
#35377=DIRECTION('ref_axis',(-0.0242942123306427,0.0709171961136464,0.997186312853627));
#35378=DIRECTION('',(0.,0.,1.));
#35379=DIRECTION('center_axis',(0.,1.,0.));
#35380=DIRECTION('ref_axis',(1.,0.,0.));
#35381=DIRECTION('',(0.,0.,1.));
#35382=DIRECTION('',(-1.,0.,0.));
#35383=DIRECTION('center_axis',(-0.946028810171404,-0.324082536286173,0.));
#35384=DIRECTION('ref_axis',(-0.324082536286173,0.946028810171404,0.));
#35385=DIRECTION('',(0.,0.,1.));
#35386=DIRECTION('center_axis',(0.946028810149194,0.324082536351006,1.04940553439243E-9));
#35387=DIRECTION('ref_axis',(-0.00521156151927112,0.015213057603577,0.999870692892276));
#35388=DIRECTION('center_axis',(0.,0.,1.));
#35389=DIRECTION('ref_axis',(-0.587785252292473,0.809016994374947,0.));
#35390=DIRECTION('',(0.,0.,1.));
#35391=DIRECTION('center_axis',(0.,-1.,0.));
#35392=DIRECTION('ref_axis',(0.,0.,-1.));
#35393=DIRECTION('',(0.,0.,1.));
#35394=DIRECTION('',(1.,0.,0.));
#35395=DIRECTION('center_axis',(1.,0.,0.));
#35396=DIRECTION('ref_axis',(0.,1.,0.));
#35397=DIRECTION('',(0.,0.,1.));
#35398=DIRECTION('center_axis',(1.,0.,0.));
#35399=DIRECTION('ref_axis',(0.,0.,1.));
#35400=DIRECTION('',(0.,0.,1.));
#35401=DIRECTION('center_axis',(0.,-1.,0.));
#35402=DIRECTION('ref_axis',(0.,0.,-1.));
#35403=DIRECTION('',(0.,0.,1.));
#35404=DIRECTION('',(-1.,0.,0.));
#35405=DIRECTION('center_axis',(1.,0.,0.));
#35406=DIRECTION('ref_axis',(0.,1.,0.));
#35407=DIRECTION('',(0.,0.,1.));
#35408=DIRECTION('center_axis',(-1.,0.,0.));
#35409=DIRECTION('ref_axis',(0.,0.,1.));
#35410=DIRECTION('center_axis',(0.,1.,0.));
#35411=DIRECTION('ref_axis',(1.,0.,0.));
#35412=DIRECTION('',(0.,0.,1.));
#35413=DIRECTION('',(-1.,0.,0.));
#35414=DIRECTION('center_axis',(-1.,0.,0.));
#35415=DIRECTION('ref_axis',(0.,0.,1.));
#35416=DIRECTION('',(0.,0.,1.));
#35417=DIRECTION('center_axis',(1.,0.,0.));
#35418=DIRECTION('ref_axis',(0.,0.,1.));
#35419=DIRECTION('center_axis',(0.,1.,0.));
#35420=DIRECTION('ref_axis',(1.,0.,0.));
#35421=DIRECTION('',(-1.,0.,0.));
#35422=DIRECTION('center_axis',(0.,0.,1.));
#35423=DIRECTION('ref_axis',(0.,1.,0.));
#35424=DIRECTION('',(0.,0.,1.));
#35425=DIRECTION('center_axis',(0.,1.,0.));
#35426=DIRECTION('ref_axis',(1.,0.,0.));
#35427=DIRECTION('',(1.,0.,0.));
#35428=DIRECTION('center_axis',(-1.,0.,0.));
#35429=DIRECTION('ref_axis',(0.,0.,1.));
#65193=CARTESIAN_POINT('',(0.,0.,0.));
#65194=CARTESIAN_POINT('Origin',(-39.,0.,13.));
#65195=CARTESIAN_POINT('',(-39.,6.64643157139886,-6.78785292759886));
#65196=CARTESIAN_POINT('',(-39.,18.3139296501741,-18.4553510063741));
#65197=CARTESIAN_POINT('',(-39.,-3.32071067811503,3.17928932191503));
#65198=CARTESIAN_POINT('',(-39.,-18.4553510063741,18.3139296501741));
#65199=CARTESIAN_POINT('Origin',(-39.,0.,0.));
#65200=CARTESIAN_POINT('',(-39.,-6.78785292759886,6.64643157139886));
#65201=CARTESIAN_POINT('',(-39.,-3.32071067811503,3.17928932191503));
#65202=CARTESIAN_POINT('Origin',(-39.,0.,0.));
#65203=CARTESIAN_POINT('Origin',(-38.25,0.,0.));
#65204=CARTESIAN_POINT('',(-37.5,19.3745972392358,-19.5160185954358));
#65205=CARTESIAN_POINT('',(-37.5,-19.5160185954358,19.3745972392358));
#65206=CARTESIAN_POINT('Origin',(-37.5,0.,0.));
#65207=CARTESIAN_POINT('',(-38.25,-18.985684800905,18.844263444705));
#65208=CARTESIAN_POINT('',(-38.25,18.844263444705,-18.985684800905));
#65209=CARTESIAN_POINT('Origin',(7.,0.,13.75));
#65210=CARTESIAN_POINT('',(7.,-17.244648771018,2.97860517091918));
#65211=CARTESIAN_POINT('',(7.,-26.2865401242261,8.07884944143965));
#65212=CARTESIAN_POINT('Origin',(7.,-15.9099025767,15.9099025767));
#65213=CARTESIAN_POINT('',(7.,-26.2865401242261,-8.07884944143965));
#65214=CARTESIAN_POINT('Origin',(7.,0.,0.));
#65215=CARTESIAN_POINT('',(7.,-17.244648771018,-2.97860517091918));
#65216=CARTESIAN_POINT('Origin',(7.,-15.9099025767,-15.9099025767));
#65217=CARTESIAN_POINT('Origin',(7.,0.,0.));
#65218=CARTESIAN_POINT('Origin',(7.,0.,13.75));
#65219=CARTESIAN_POINT('',(7.,-2.97860517091918,-17.244648771018));
#65220=CARTESIAN_POINT('',(7.,-8.07884944143965,-26.2865401242261));
#65221=CARTESIAN_POINT('Origin',(7.,-15.9099025767,-15.9099025767));
#65222=CARTESIAN_POINT('',(7.,8.07884944143965,-26.2865401242261));
#65223=CARTESIAN_POINT('Origin',(7.,0.,0.));
#65224=CARTESIAN_POINT('',(7.,2.97860517091918,-17.244648771018));
#65225=CARTESIAN_POINT('Origin',(7.,15.9099025767,-15.9099025767));
#65226=CARTESIAN_POINT('Origin',(7.,0.,0.));
#65227=CARTESIAN_POINT('Origin',(-1.,0.,0.));
#65228=CARTESIAN_POINT('',(-9.,2.97860517091918,-17.244648771018));
#65229=CARTESIAN_POINT('',(-9.,-2.97860517091918,-17.244648771018));
#65230=CARTESIAN_POINT('Origin',(-9.,0.,0.));
#65231=CARTESIAN_POINT('',(-1.,-2.97860517091918,-17.244648771018));
#65232=CARTESIAN_POINT('',(-1.,2.97860517091918,-17.244648771018));
#65233=CARTESIAN_POINT('Origin',(-1.,0.,0.));
#65234=CARTESIAN_POINT('',(-9.,-17.244648771018,2.97860517091918));
#65235=CARTESIAN_POINT('',(-1.,-17.244648771018,2.97860517091918));
#65236=CARTESIAN_POINT('',(-9.,-17.244648771018,-2.97860517091918));
#65237=CARTESIAN_POINT('',(-1.,-17.244648771018,-2.97860517091918));
#65238=CARTESIAN_POINT('Origin',(-9.,0.,0.));
#65239=CARTESIAN_POINT('Origin',(-1.,15.9099025767,-15.9099025767));
#65240=CARTESIAN_POINT('',(-9.,8.07884944143965,-26.2865401242261));
#65241=CARTESIAN_POINT('',(-1.,8.07884944143965,-26.2865401242261));
#65242=CARTESIAN_POINT('Origin',(-9.,15.9099025767,-15.9099025767));
#65243=CARTESIAN_POINT('Origin',(-1.,-15.9099025767,-15.9099025767));
#65244=CARTESIAN_POINT('',(-9.,-26.2865401242261,-8.07884944143965));
#65245=CARTESIAN_POINT('',(-1.,-26.2865401242261,-8.07884944143965));
#65246=CARTESIAN_POINT('Origin',(-9.,-15.9099025767,-15.9099025767));
#65247=CARTESIAN_POINT('Origin',(-1.,-15.9099025767,-15.9099025767));
#65248=CARTESIAN_POINT('',(-9.,-8.07884944143965,-26.2865401242261));
#65249=CARTESIAN_POINT('Origin',(-9.,-15.9099025767,-15.9099025767));
#65250=CARTESIAN_POINT('',(-1.,-8.07884944143965,-26.2865401242261));
#65251=CARTESIAN_POINT('Origin',(-1.,-15.9099025767,15.9099025767));
#65252=CARTESIAN_POINT('',(-9.,-26.2865401242261,8.07884944143965));
#65253=CARTESIAN_POINT('Origin',(-9.,-15.9099025767,15.9099025767));
#65254=CARTESIAN_POINT('',(-1.,-26.2865401242261,8.07884944143965));
#65255=CARTESIAN_POINT('Origin',(-15.25,0.,0.));
#65256=CARTESIAN_POINT('Origin',(-9.,0.,0.));
#65257=CARTESIAN_POINT('',(-9.,-19.5160185954358,19.3745972392358));
#65258=CARTESIAN_POINT('Origin',(-9.,0.,0.));
#65259=CARTESIAN_POINT('',(-15.25,-19.5160185954358,19.3745972392358));
#65260=CARTESIAN_POINT('',(-9.,19.3745972392358,-19.5160185954358));
#65261=CARTESIAN_POINT('',(-15.25,19.3745972392358,-19.5160185954358));
#65262=CARTESIAN_POINT('Origin',(-9.,0.,0.));
#65263=CARTESIAN_POINT('',(-26.4377160017629,5.20014826788293E-15,-27.5));
#65264=CARTESIAN_POINT('',(-21.5,0.795787808628117,-27.4884834387719));
#65265=CARTESIAN_POINT('Ctrl Pts',(-26.4377160017635,3.62918028962156E-12,
-27.5));
#65266=CARTESIAN_POINT('Ctrl Pts',(-26.4059901055898,-0.197224429757389,
-27.5));
#65267=CARTESIAN_POINT('Ctrl Pts',(-26.3612673723093,-0.394306822151656,
-27.4978432541329));
#65268=CARTESIAN_POINT('Ctrl Pts',(-26.1640017219763,-1.04038440540881,
-27.4840667670191));
#65269=CARTESIAN_POINT('Ctrl Pts',(-25.9451630528242,-1.46536445881011,
-27.4630238360419));
#65270=CARTESIAN_POINT('Ctrl Pts',(-25.4583216143471,-2.03730160051001,
-27.4254298732512));
#65271=CARTESIAN_POINT('Ctrl Pts',(-25.2031277311753,-2.25352124915401,
-27.4079090802056));
#65272=CARTESIAN_POINT('Ctrl Pts',(-24.6276828245851,-2.54794284417893,
-27.3821077345433));
#65273=CARTESIAN_POINT('Ctrl Pts',(-24.3071450917694,-2.62563132929186,
-27.3743686707592));
#65274=CARTESIAN_POINT('Ctrl Pts',(-23.6928549082306,-2.62563132929186,
-27.3743686707592));
#65275=CARTESIAN_POINT('Ctrl Pts',(-23.3723171754149,-2.54794284417893,
-27.3821077345433));
#65276=CARTESIAN_POINT('Ctrl Pts',(-22.7968722688247,-2.25352124915401,
-27.4079090802056));
#65277=CARTESIAN_POINT('Ctrl Pts',(-22.5416783856529,-2.03730160051001,
-27.4254298732512));
#65278=CARTESIAN_POINT('Ctrl Pts',(-22.0548369471758,-1.46536445881011,
-27.4630238360419));
#65279=CARTESIAN_POINT('Ctrl Pts',(-21.8359982780237,-1.04038440540881,
-27.4840667670191));
#65280=CARTESIAN_POINT('Ctrl Pts',(-21.5586819382303,-0.132127593799674,
-27.5034337727556));
#65281=CARTESIAN_POINT('Ctrl Pts',(-21.5,0.351095281866489,-27.501357226159));
#65282=CARTESIAN_POINT('Ctrl Pts',(-21.5,0.795787808628117,-27.4884834387719));
#65283=CARTESIAN_POINT('Ctrl Pts',(-21.5,0.795787808628117,-27.4884834387719));
#65284=CARTESIAN_POINT('Ctrl Pts',(-21.5,1.29514612764106,-27.4740270842301));
#65285=CARTESIAN_POINT('Ctrl Pts',(-21.5732810359516,1.83467613548264,-27.4435694082118));
#65286=CARTESIAN_POINT('Ctrl Pts',(-21.875132610179,2.86152046064611,-27.3555705260108));
#65287=CARTESIAN_POINT('Ctrl Pts',(-22.1019786827804,3.34936228446823,-27.2982789021101));
#65288=CARTESIAN_POINT('Ctrl Pts',(-22.5800189982867,4.00649576099619,-27.2078036326968));
#65289=CARTESIAN_POINT('Ctrl Pts',(-22.8176675360951,4.25837971422122,-27.1689143482003));
#65290=CARTESIAN_POINT('Ctrl Pts',(-23.230437709971,4.53014788237278,-27.1244573394495));
#65291=CARTESIAN_POINT('Ctrl Pts',(-23.3774232617091,4.60348624022732,-27.1119971008064));
#65292=CARTESIAN_POINT('Ctrl Pts',(-23.6826872283767,4.70319063996839,-27.0948822448621));
#65293=CARTESIAN_POINT('Ctrl Pts',(-23.8409645128472,4.72956268912345,-27.0902424642094));
#65294=CARTESIAN_POINT('Ctrl Pts',(-24.,4.72956268912345,-27.0902424642094));
#65295=CARTESIAN_POINT('Ctrl Pts',(-24.1590354871528,4.72956268912345,-27.0902424642094));
#65296=CARTESIAN_POINT('Ctrl Pts',(-24.3173127716233,4.70319063996839,-27.0948822448621));
#65297=CARTESIAN_POINT('Ctrl Pts',(-24.6225767382909,4.60348624022732,-27.1119971008064));
#65298=CARTESIAN_POINT('Ctrl Pts',(-24.769562290029,4.53014788237278,-27.1244573394495));
#65299=CARTESIAN_POINT('Ctrl Pts',(-25.1823324639049,4.25837971422122,-27.1689143482003));
#65300=CARTESIAN_POINT('Ctrl Pts',(-25.4199810017133,4.00649576099619,-27.2078036326968));
#65301=CARTESIAN_POINT('Ctrl Pts',(-25.8980213172196,3.34936228446823,-27.2982789021101));
#65302=CARTESIAN_POINT('Ctrl Pts',(-26.124867389821,2.86152046064611,-27.3555705260108));
#65303=CARTESIAN_POINT('Ctrl Pts',(-26.4267189640484,1.83467613548264,-27.4435694082118));
#65304=CARTESIAN_POINT('Ctrl Pts',(-26.5,1.29514612764106,-27.4740270842301));
#65305=CARTESIAN_POINT('Ctrl Pts',(-26.5,0.539056139721172,-27.4959157852184));
#65306=CARTESIAN_POINT('Ctrl Pts',(-26.4810497169061,0.269384581345093,
-27.5));
#65307=CARTESIAN_POINT('Ctrl Pts',(-26.4377160017635,3.62852109470069E-12,
-27.5));
#65308=CARTESIAN_POINT('',(-26.7834228083186,-25.9817095809707,9.0111468332335));
#65309=CARTESIAN_POINT('',(-21.2165771916814,-25.9817095809707,9.01114683323349));
#65310=CARTESIAN_POINT('',(-24.,-25.9817095809707,9.01114683323349));
#65311=CARTESIAN_POINT('Ctrl Pts',(-21.2165771916814,-25.9817095809707,
9.01114683323346));
#65312=CARTESIAN_POINT('Ctrl Pts',(-20.9800185929094,-26.0859415162294,
8.71061639897562));
#65313=CARTESIAN_POINT('Ctrl Pts',(-20.7644137903678,-26.1896244767548,
8.39410853029323));
#65314=CARTESIAN_POINT('Ctrl Pts',(-19.9481928010943,-26.5980125778779,
7.06565470065933));
#65315=CARTESIAN_POINT('Ctrl Pts',(-19.4277281498739,-26.8979580454901,
5.86356256779912));
#65316=CARTESIAN_POINT('Ctrl Pts',(-18.7008421968423,-27.3256746578734,
3.34500173130744));
#65317=CARTESIAN_POINT('Ctrl Pts',(-18.5,-27.4528451038414,2.02682423429658));
#65318=CARTESIAN_POINT('Ctrl Pts',(-18.5,-27.5154319978194,-0.135082218585487));
#65319=CARTESIAN_POINT('Ctrl Pts',(-18.6175304465915,-27.4923164791461,
-1.14719857365593));
#65320=CARTESIAN_POINT('Ctrl Pts',(-19.2063453548323,-27.3486548092588,
-3.0322593031978));
#65321=CARTESIAN_POINT('Ctrl Pts',(-19.6800566608577,-27.230211420678,-3.90460446975071));
#65322=CARTESIAN_POINT('Ctrl Pts',(-20.7520277927271,-27.0309364869423,
-5.08230700100516));
#65323=CARTESIAN_POINT('Ctrl Pts',(-21.328545241257,-26.9408345358146,-5.5257234492484));
#65324=CARTESIAN_POINT('Ctrl Pts',(-22.6156966073873,-26.8122687238307,
-6.11918487834519));
#65325=CARTESIAN_POINT('Ctrl Pts',(-23.3263251783663,-26.7757599690515,
-6.26966331470342));
#65326=CARTESIAN_POINT('Ctrl Pts',(-24.6736748216337,-26.7757599690515,
-6.26966331470342));
#65327=CARTESIAN_POINT('Ctrl Pts',(-25.3843033926127,-26.8122687238307,
-6.11918487834519));
#65328=CARTESIAN_POINT('Ctrl Pts',(-26.671454758743,-26.9408345358146,-5.5257234492484));
#65329=CARTESIAN_POINT('Ctrl Pts',(-27.2479722072729,-27.0309364869423,
-5.08230700100516));
#65330=CARTESIAN_POINT('Ctrl Pts',(-28.3199433391423,-27.230211420678,-3.90460446975071));
#65331=CARTESIAN_POINT('Ctrl Pts',(-28.7936546451677,-27.3486548092588,
-3.0322593031978));
#65332=CARTESIAN_POINT('Ctrl Pts',(-29.3824695534085,-27.4923164791461,
-1.14719857365593));
#65333=CARTESIAN_POINT('Ctrl Pts',(-29.5,-27.5154319978194,-0.135082218585487));
#65334=CARTESIAN_POINT('Ctrl Pts',(-29.5,-27.4528451038414,2.02682423429658));
#65335=CARTESIAN_POINT('Ctrl Pts',(-29.2991578031577,-27.3256746578734,
3.34500173130745));
#65336=CARTESIAN_POINT('Ctrl Pts',(-28.5722718501261,-26.8979580454901,
5.86356256779912));
#65337=CARTESIAN_POINT('Ctrl Pts',(-28.0518071989057,-26.5980125778779,
7.06565470065933));
#65338=CARTESIAN_POINT('Ctrl Pts',(-27.2355862096322,-26.1896244767548,
8.39410853029323));
#65339=CARTESIAN_POINT('Ctrl Pts',(-27.0199814070906,-26.0859415162294,
8.71061639897562));
#65340=CARTESIAN_POINT('Ctrl Pts',(-26.7834228083186,-25.9817095809707,
9.01114683323346));
#65341=CARTESIAN_POINT('Origin',(-24.,0.,0.));
#65342=CARTESIAN_POINT('',(-9.,-6.78785292759886,6.64643157139886));
#65343=CARTESIAN_POINT('',(-24.,-6.78785292759886,6.64643157139886));
#65344=CARTESIAN_POINT('',(-9.,6.64643157139886,-6.78785292759886));
#65345=CARTESIAN_POINT('Origin',(-9.,0.,0.));
#65346=CARTESIAN_POINT('',(-24.,6.64643157139886,-6.78785292759886));
#65347=CARTESIAN_POINT('Origin',(-9.,15.9099025767,-15.9099025767));
#65348=CARTESIAN_POINT('',(-9.,7.88424061023497,-8.02566196643497));
#65349=CARTESIAN_POINT('',(-9.,7.88424061023497,-8.02566196643497));
#65350=CARTESIAN_POINT('Origin',(-24.,5.48007755379487,-22.8041936936052));
#65351=CARTESIAN_POINT('',(-21.5,14.0714249456,-14.2128463018001));
#65352=CARTESIAN_POINT('',(-21.5,5.48007755379487,-22.8041936936052));
#65353=CARTESIAN_POINT('Origin',(-24.,14.0714249456,-14.2128463018001));
#65354=CARTESIAN_POINT('Origin',(-28.4,-22.6274169975687,5.65685424983145));
#65355=CARTESIAN_POINT('Origin',(-24.,-22.6274169975687,5.65685424983145));
#65356=CARTESIAN_POINT('',(-20.7,-22.6274169975687,5.65685424983145));
#65357=CARTESIAN_POINT('Origin',(-24.,-22.6274169975687,5.65685424983145));
#65358=CARTESIAN_POINT('Origin',(-24.,-19.4454364822292,8.8388347651709));
#65359=CARTESIAN_POINT('',(-20.7,-16.2634559668898,12.0208152805104));
#65360=CARTESIAN_POINT('Origin',(-24.,-16.2634559668898,12.0208152805104));
#65361=CARTESIAN_POINT('',(-20.7,-19.4454364822292,8.8388347651709));
#65362=CARTESIAN_POINT('Origin',(-26.9,-16.2634559668898,12.0208152805104));
#65363=CARTESIAN_POINT('',(-21.5,-16.2634559668898,12.0208152805104));
#65364=CARTESIAN_POINT('Origin',(-24.,-16.2634559668898,12.0208152805104));
#65365=CARTESIAN_POINT('Origin',(-24.,-5.48007755379487,22.8041936936052));
#65366=CARTESIAN_POINT('',(-21.5,-14.2128463018,14.0714249456001));
#65367=CARTESIAN_POINT('Origin',(-24.,-14.2128463018,14.0714249456001));
#65368=CARTESIAN_POINT('',(-21.5,-5.48007755379487,22.8041936936052));
#65369=CARTESIAN_POINT('Origin',(-16.,-0.070710678130059,-0.0707106780699435));
#65370=CARTESIAN_POINT('Origin',(-16.,-0.070710678130059,-0.0707106780699435));
#65371=CARTESIAN_POINT('Origin',(-24.,-28.1074945517644,0.176776695635716));
#65372=CARTESIAN_POINT('Origin',(-24.,28.1074945517644,-0.176776695635716));
#65373=CARTESIAN_POINT('',(-26.7834228083186,25.9817095809707,-9.0111468332335));
#65374=CARTESIAN_POINT('',(-21.2165771916814,25.9817095809707,-9.01114683323349));
#65375=CARTESIAN_POINT('Origin',(-24.,22.6274169975687,-5.65685424983145));
#65376=CARTESIAN_POINT('Ctrl Pts',(-26.7834228083186,25.9817095809707,-9.01114683323346));
#65377=CARTESIAN_POINT('Ctrl Pts',(-27.0199814070906,26.0859415162294,-8.71061639897562));
#65378=CARTESIAN_POINT('Ctrl Pts',(-27.2355862096322,26.1896244767548,-8.39410853029323));
#65379=CARTESIAN_POINT('Ctrl Pts',(-28.0518071989057,26.5980125778779,-7.06565470065933));
#65380=CARTESIAN_POINT('Ctrl Pts',(-28.5722718501261,26.8979580454901,-5.86356256779912));
#65381=CARTESIAN_POINT('Ctrl Pts',(-29.2991578031577,27.3256746578734,-3.34500173130745));
#65382=CARTESIAN_POINT('Ctrl Pts',(-29.5,27.4528451038414,-2.02682423429658));
#65383=CARTESIAN_POINT('Ctrl Pts',(-29.5,27.5154319978194,0.135082218585487));
#65384=CARTESIAN_POINT('Ctrl Pts',(-29.3824695534085,27.4923164791461,1.14719857365593));
#65385=CARTESIAN_POINT('Ctrl Pts',(-28.7936546451677,27.3486548092588,3.0322593031978));
#65386=CARTESIAN_POINT('Ctrl Pts',(-28.3199433391423,27.230211420678,3.90460446975071));
#65387=CARTESIAN_POINT('Ctrl Pts',(-27.2479722072729,27.0309364869423,5.08230700100516));
#65388=CARTESIAN_POINT('Ctrl Pts',(-26.671454758743,26.9408345358146,5.5257234492484));
#65389=CARTESIAN_POINT('Ctrl Pts',(-25.3843033926127,26.8122687238307,6.11918487834519));
#65390=CARTESIAN_POINT('Ctrl Pts',(-24.6736748216337,26.7757599690515,6.26966331470342));
#65391=CARTESIAN_POINT('Ctrl Pts',(-23.3263251783663,26.7757599690515,6.26966331470342));
#65392=CARTESIAN_POINT('Ctrl Pts',(-22.6156966073873,26.8122687238307,6.11918487834518));
#65393=CARTESIAN_POINT('Ctrl Pts',(-21.328545241257,26.9408345358146,5.52572344924839));
#65394=CARTESIAN_POINT('Ctrl Pts',(-20.7520277927271,27.0309364869423,5.08230700100516));
#65395=CARTESIAN_POINT('Ctrl Pts',(-19.6800566608577,27.230211420678,3.90460446975071));
#65396=CARTESIAN_POINT('Ctrl Pts',(-19.2063453548323,27.3486548092588,3.0322593031978));
#65397=CARTESIAN_POINT('Ctrl Pts',(-18.6175304465915,27.4923164791461,1.14719857365593));
#65398=CARTESIAN_POINT('Ctrl Pts',(-18.5,27.5154319978194,0.135082218585486));
#65399=CARTESIAN_POINT('Ctrl Pts',(-18.5,27.4528451038414,-2.02682423429658));
#65400=CARTESIAN_POINT('Ctrl Pts',(-18.7008421968423,27.3256746578734,-3.34500173130745));
#65401=CARTESIAN_POINT('Ctrl Pts',(-19.4277281498739,26.8979580454901,-5.86356256779912));
#65402=CARTESIAN_POINT('Ctrl Pts',(-19.9481928010943,26.5980125778779,-7.06565470065933));
#65403=CARTESIAN_POINT('Ctrl Pts',(-20.7644137903678,26.1896244767548,-8.39410853029323));
#65404=CARTESIAN_POINT('Ctrl Pts',(-20.9800185929094,26.0859415162294,-8.71061639897562));
#65405=CARTESIAN_POINT('Ctrl Pts',(-21.2165771916814,25.9817095809707,-9.01114683323346));
#65406=CARTESIAN_POINT('Origin',(-16.,0.0707106781072506,0.070710678167366));
#65407=CARTESIAN_POINT('',(-39.,-18.3139296501367,18.4553510064113));
#65408=CARTESIAN_POINT('',(-37.5,-19.3745972391984,19.516018595473));
#65409=CARTESIAN_POINT('',(-38.25,-18.8442634446675,18.9856848009421));
#65410=CARTESIAN_POINT('',(-39.,-6.64643157136116,6.78785292763578));
#65411=CARTESIAN_POINT('',(-39.,-3.17928932187772,3.32071067815234));
#65412=CARTESIAN_POINT('',(-9.,-6.64643157136116,6.78785292763578));
#65413=CARTESIAN_POINT('',(-24.,-6.64643157136116,6.78785292763578));
#65414=CARTESIAN_POINT('',(-9.,-19.3745972391984,19.516018595473));
#65415=CARTESIAN_POINT('',(-9.,8.02566196647228,-7.88424061019766));
#65416=CARTESIAN_POINT('',(-15.25,-19.3745972391984,19.516018595473));
#65417=CARTESIAN_POINT('',(-21.5,-14.0714249455627,14.2128463018374));
#65418=CARTESIAN_POINT('Origin',(-24.,-14.0714249455627,14.2128463018374));
#65419=CARTESIAN_POINT('Origin',(-24.,-5.48007755379487,22.8041936936052));
#65420=CARTESIAN_POINT('',(-24.,-4.72956268912343,27.0902424642094));
#65421=CARTESIAN_POINT('',(-21.5,-0.795787808628118,27.4884834387719));
#65422=CARTESIAN_POINT('Ctrl Pts',(-21.5,-0.795787808628116,27.4884834387719));
#65423=CARTESIAN_POINT('Ctrl Pts',(-21.5,-0.351095281866489,27.501357226159));
#65424=CARTESIAN_POINT('Ctrl Pts',(-21.5586819382303,0.132127593799674,
27.5034337727556));
#65425=CARTESIAN_POINT('Ctrl Pts',(-21.8359982780237,1.04038440540881,27.4840667670191));
#65426=CARTESIAN_POINT('Ctrl Pts',(-22.0548369471758,1.46536445881011,27.4630238360419));
#65427=CARTESIAN_POINT('Ctrl Pts',(-22.5416783856529,2.03730160051001,27.4254298732512));
#65428=CARTESIAN_POINT('Ctrl Pts',(-22.7968722688247,2.25352124915401,27.4079090802056));
#65429=CARTESIAN_POINT('Ctrl Pts',(-23.3723171754149,2.54794284417893,27.3821077345433));
#65430=CARTESIAN_POINT('Ctrl Pts',(-23.6928549082306,2.62563132929186,27.3743686707592));
#65431=CARTESIAN_POINT('Ctrl Pts',(-24.3071450917694,2.62563132929186,27.3743686707592));
#65432=CARTESIAN_POINT('Ctrl Pts',(-24.6276828245851,2.54794284417893,27.3821077345433));
#65433=CARTESIAN_POINT('Ctrl Pts',(-25.2031277311753,2.25352124915401,27.4079090802056));
#65434=CARTESIAN_POINT('Ctrl Pts',(-25.4583216143471,2.03730160051001,27.4254298732512));
#65435=CARTESIAN_POINT('Ctrl Pts',(-25.9451630528242,1.46536445881011,27.4630238360419));
#65436=CARTESIAN_POINT('Ctrl Pts',(-26.1640017219763,1.04038440540881,27.4840667670191));
#65437=CARTESIAN_POINT('Ctrl Pts',(-26.4413180617697,0.132127593799674,
27.5034337727556));
#65438=CARTESIAN_POINT('Ctrl Pts',(-26.5,-0.351095281866489,27.501357226159));
#65439=CARTESIAN_POINT('Ctrl Pts',(-26.5,-1.29514612764106,27.4740270842301));
#65440=CARTESIAN_POINT('Ctrl Pts',(-26.4267189640484,-1.83467613548264,
27.4435694082118));
#65441=CARTESIAN_POINT('Ctrl Pts',(-26.124867389821,-2.86152046064611,27.3555705260108));
#65442=CARTESIAN_POINT('Ctrl Pts',(-25.8980213172196,-3.34936228446823,
27.2982789021101));
#65443=CARTESIAN_POINT('Ctrl Pts',(-25.4199810017133,-4.00649576099619,
27.2078036326968));
#65444=CARTESIAN_POINT('Ctrl Pts',(-25.1823324639049,-4.25837971422122,
27.1689143482003));
#65445=CARTESIAN_POINT('Ctrl Pts',(-24.769562290029,-4.53014788237278,27.1244573394495));
#65446=CARTESIAN_POINT('Ctrl Pts',(-24.6225767382909,-4.60348624022732,
27.1119971008064));
#65447=CARTESIAN_POINT('Ctrl Pts',(-24.3173127716233,-4.70319063996839,
27.0948822448621));
#65448=CARTESIAN_POINT('Ctrl Pts',(-24.1590354871528,-4.72956268912345,
27.0902424642093));
#65449=CARTESIAN_POINT('Ctrl Pts',(-24.,-4.72956268912345,27.0902424642093));
#65450=CARTESIAN_POINT('Ctrl Pts',(-24.,-4.72956268912345,27.0902424642093));
#65451=CARTESIAN_POINT('Ctrl Pts',(-23.8409645128472,-4.72956268912345,
27.0902424642093));
#65452=CARTESIAN_POINT('Ctrl Pts',(-23.6826872283767,-4.70319063996839,
27.0948822448621));
#65453=CARTESIAN_POINT('Ctrl Pts',(-23.3774232617091,-4.60348624022732,
27.1119971008064));
#65454=CARTESIAN_POINT('Ctrl Pts',(-23.230437709971,-4.53014788237278,27.1244573394495));
#65455=CARTESIAN_POINT('Ctrl Pts',(-22.8176675360951,-4.25837971422122,
27.1689143482003));
#65456=CARTESIAN_POINT('Ctrl Pts',(-22.5800189982867,-4.00649576099619,
27.2078036326968));
#65457=CARTESIAN_POINT('Ctrl Pts',(-22.1019786827804,-3.34936228446823,
27.2982789021101));
#65458=CARTESIAN_POINT('Ctrl Pts',(-21.875132610179,-2.86152046064611,27.3555705260108));
#65459=CARTESIAN_POINT('Ctrl Pts',(-21.5732810359516,-1.83467613548264,
27.4435694082118));
#65460=CARTESIAN_POINT('Ctrl Pts',(-21.5,-1.29514612764106,27.4740270842301));
#65461=CARTESIAN_POINT('Ctrl Pts',(-21.5,-0.795787808628117,27.4884834387719));
#65462=CARTESIAN_POINT('',(-21.5,-5.48007755379487,22.8041936936052));
#65463=CARTESIAN_POINT('Origin',(-24.,5.48007755379487,-22.8041936936052));
#65464=CARTESIAN_POINT('',(-21.5,14.2128463018373,-14.0714249455628));
#65465=CARTESIAN_POINT('Origin',(-24.,14.2128463018373,-14.0714249455628));
#65466=CARTESIAN_POINT('',(-21.5,16.2634559668897,-12.0208152805104));
#65467=CARTESIAN_POINT('',(-21.5,5.48007755379487,-22.8041936936052));
#65468=CARTESIAN_POINT('Origin',(-24.,16.2634559668898,-12.0208152805104));
#65469=CARTESIAN_POINT('Origin',(-26.9,16.2634559668898,-12.0208152805104));
#65470=CARTESIAN_POINT('',(-20.7,16.2634559668898,-12.0208152805104));
#65471=CARTESIAN_POINT('Origin',(-24.,16.2634559668898,-12.0208152805104));
#65472=CARTESIAN_POINT('Origin',(-24.,19.4454364822292,-8.8388347651709));
#65473=CARTESIAN_POINT('',(-20.7,22.6274169975687,-5.65685424983145));
#65474=CARTESIAN_POINT('',(-20.7,19.4454364822292,-8.8388347651709));
#65475=CARTESIAN_POINT('Origin',(-24.,22.6274169975687,-5.65685424983145));
#65476=CARTESIAN_POINT('Origin',(-28.4,22.6274169975687,-5.65685424983145));
#65477=CARTESIAN_POINT('',(-24.,25.9817095809707,-9.01114683323349));
#65478=CARTESIAN_POINT('Origin',(-16.,0.0707106781072506,0.070710678167366));
#65479=CARTESIAN_POINT('',(-37.5,19.516018595473,-19.3745972391984));
#65480=CARTESIAN_POINT('',(-39.,18.4553510064113,-18.3139296501367));
#65481=CARTESIAN_POINT('',(-38.25,18.9856848009421,-18.8442634446675));
#65482=CARTESIAN_POINT('',(-9.,19.516018595473,-19.3745972391984));
#65483=CARTESIAN_POINT('',(-15.25,19.516018595473,-19.3745972391984));
#65484=CARTESIAN_POINT('',(-9.,6.78785292763578,-6.64643157136116));
#65485=CARTESIAN_POINT('',(-9.,8.02566196647228,-7.88424061019766));
#65486=CARTESIAN_POINT('',(-39.,6.78785292763578,-6.64643157136116));
#65487=CARTESIAN_POINT('',(-24.,6.78785292763578,-6.64643157136116));
#65488=CARTESIAN_POINT('',(-39.,-3.17928932187772,3.32071067815234));
#65489=CARTESIAN_POINT('Origin',(-39.,0.,13.));
#65490=CARTESIAN_POINT('',(-39.,8.4950947355237,4.25245404848513));
#65491=CARTESIAN_POINT('Origin',(-39.,0.,0.));
#65492=CARTESIAN_POINT('',(-39.,10.8187337521138,6.57609306507525));
#65493=CARTESIAN_POINT('',(-39.,7.54567369566792,3.30303300862935));
#65494=CARTESIAN_POINT('',(-39.,6.57609306499454,10.8187337521945));
#65495=CARTESIAN_POINT('',(-39.,5.44741340857436,11.9474134086147));
#65496=CARTESIAN_POINT('',(-39.,4.25245404837755,8.49509473557755));
#65497=CARTESIAN_POINT('',(-39.,3.30303300854864,7.54567369574863));
#65498=CARTESIAN_POINT('Origin',(-39.,0.,0.));
#65499=CARTESIAN_POINT('Origin',(-39.,0.,0.));
#65500=CARTESIAN_POINT('Origin',(-38.25,0.,0.));
#65501=CARTESIAN_POINT('Origin',(-37.5,0.,0.));
#65502=CARTESIAN_POINT('Origin',(-9.,15.9099025767,-15.9099025767));
#65503=CARTESIAN_POINT('',(-9.,26.2865401242261,-8.07884944143965));
#65504=CARTESIAN_POINT('Origin',(-9.,0.,0.));
#65505=CARTESIAN_POINT('',(-9.,17.244648771018,-2.97860517091918));
#65506=CARTESIAN_POINT('Origin',(-9.,15.9099025767,-15.9099025767));
#65507=CARTESIAN_POINT('',(-9.,17.244648771018,2.97860517091918));
#65508=CARTESIAN_POINT('Origin',(-9.,0.,0.));
#65509=CARTESIAN_POINT('',(-9.,26.2865401242261,8.07884944143965));
#65510=CARTESIAN_POINT('Origin',(-9.,15.9099025767,15.9099025767));
#65511=CARTESIAN_POINT('',(-9.,8.07884944143965,26.2865401242261));
#65512=CARTESIAN_POINT('Origin',(-9.,0.,0.));
#65513=CARTESIAN_POINT('',(-9.,2.97860517091918,17.244648771018));
#65514=CARTESIAN_POINT('Origin',(-9.,15.9099025767,15.9099025767));
#65515=CARTESIAN_POINT('',(-9.,-2.97860517091918,17.244648771018));
#65516=CARTESIAN_POINT('Origin',(-9.,0.,0.));
#65517=CARTESIAN_POINT('',(-9.,-8.07884944143965,26.2865401242261));
#65518=CARTESIAN_POINT('Origin',(-9.,-15.9099025767,15.9099025767));
#65519=CARTESIAN_POINT('Origin',(-9.,0.,0.));
#65520=CARTESIAN_POINT('',(-9.,4.25245404837755,8.49509473557755));
#65521=CARTESIAN_POINT('Origin',(-9.,0.,0.));
#65522=CARTESIAN_POINT('',(-9.,6.57609306499454,10.8187337521945));
#65523=CARTESIAN_POINT('',(-9.,0.0530330085486312,4.29567369574864));
#65524=CARTESIAN_POINT('',(-9.,10.8187337521138,6.57609306507525));
#65525=CARTESIAN_POINT('',(-9.,16.6523646969244,0.742462120264717));
#65526=CARTESIAN_POINT('',(-9.,8.4950947355237,4.25245404848513));
#65527=CARTESIAN_POINT('',(-9.,4.29567369566792,0.0530330086293516));
#65528=CARTESIAN_POINT('Origin',(-9.,0.,0.));
#65529=CARTESIAN_POINT('Origin',(-24.,0.,0.));
#65530=CARTESIAN_POINT('',(-24.,4.25245404837755,8.49509473557755));
#65531=CARTESIAN_POINT('Origin',(-24.,0.,0.));
#65532=CARTESIAN_POINT('',(-24.,8.4950947355237,4.25245404848513));
#65533=CARTESIAN_POINT('Origin',(-15.25,0.,0.));
#65534=CARTESIAN_POINT('',(-3.7202200813,-0.2994444445,27.498369643029));
#65535=CARTESIAN_POINT('',(-4.3435534146,-0.2994444445,27.498369643029));
#65536=CARTESIAN_POINT('',(-4.03188674795,-0.2994444445,27.498369643029));
#65537=CARTESIAN_POINT('',(-4.3435534146,-1.1061111111,27.4777458720671));
#65538=CARTESIAN_POINT('Ctrl Pts',(-4.3435534146,-0.2994444445,27.498369643029));
#65539=CARTESIAN_POINT('Ctrl Pts',(-4.39419602744118,-0.2994444445,27.498369643029));
#65540=CARTESIAN_POINT('Ctrl Pts',(-4.44821405117923,-0.309565273785878,
27.4982652712794));
#65541=CARTESIAN_POINT('Ctrl Pts',(-4.54758440972013,-0.350724834122933,
27.4977711038395));
#65542=CARTESIAN_POINT('Ctrl Pts',(-4.59293670765284,-0.381763557784472,
27.4973733109335));
#65543=CARTESIAN_POINT('Ctrl Pts',(-4.66456223528332,-0.453385171307823,
27.4962856562635));
#65544=CARTESIAN_POINT('Ctrl Pts',(-4.69560557365306,-0.498744419672721,
27.4955218892374));
#65545=CARTESIAN_POINT('Ctrl Pts',(-4.7367677324877,-0.598121989127674,
27.493539605584));
#65546=CARTESIAN_POINT('Ctrl Pts',(-4.7468867479,-0.652140069806569,27.4923130926182));
#65547=CARTESIAN_POINT('Ctrl Pts',(-4.7468867479,-0.753430235839141,27.4897237204729));
#65548=CARTESIAN_POINT('Ctrl Pts',(-4.73676246101481,-0.80745512421137,
27.4881881502515));
#65549=CARTESIAN_POINT('Ctrl Pts',(-4.69559144465381,-0.906836412476876,
27.4850890353706));
#65550=CARTESIAN_POINT('Ctrl Pts',(-4.66454479714166,-0.952193095307298,
27.4835334801247));
#65551=CARTESIAN_POINT('Ctrl Pts',(-4.59292152712871,-1.0238019031852,27.4809590925011));
#65552=CARTESIAN_POINT('Ctrl Pts',(-4.54757596140155,-1.054834879545,27.479769785307));
#65553=CARTESIAN_POINT('Ctrl Pts',(-4.44821406584017,-1.09598961694164,
27.4781591602539));
#65554=CARTESIAN_POINT('Ctrl Pts',(-4.39419749547155,-1.1061111111,27.4777458720671));
#65555=CARTESIAN_POINT('Ctrl Pts',(-4.3435534146,-1.1061111111,27.4777458720671));
#65556=CARTESIAN_POINT('',(-3.7202200813,-1.1061111111,27.4777458720671));
#65557=CARTESIAN_POINT('',(-4.03188674795,-1.1061111111,27.4777458720671));
#65558=CARTESIAN_POINT('Origin',(-3.7202200813,0.,0.));
#65559=CARTESIAN_POINT('Origin',(-29.,9.72271824131503,9.72271824131503));
#65560=CARTESIAN_POINT('',(-31.1,8.69741340859454,8.69741340859454));
#65561=CARTESIAN_POINT('Origin',(-29.,8.69741340859454,8.69741340859454));
#65562=CARTESIAN_POINT('',(-31.1,19.4454364826301,19.4454364826301));
#65563=CARTESIAN_POINT('',(-31.1,9.72271824131503,9.72271824131503));
#65564=CARTESIAN_POINT('',(-26.9,19.4454364826301,19.4454364826301));
#65565=CARTESIAN_POINT('Ctrl Pts',(-26.9,19.4454364826301,19.4454364826301));
#65566=CARTESIAN_POINT('Ctrl Pts',(-26.9,19.2589082724023,19.6319646928578));
#65567=CARTESIAN_POINT('Ctrl Pts',(-26.9527396524836,19.0570372826678,19.827917294343));
#65568=CARTESIAN_POINT('Ctrl Pts',(-27.167084371912,18.6805067132861,20.1830533656328));
#65569=CARTESIAN_POINT('Ctrl Pts',(-27.3286837627136,18.5059934629633,20.3423953731785));
#65570=CARTESIAN_POINT('Ctrl Pts',(-27.7014679712018,18.2281408464247,20.5917392401225));
#65571=CARTESIAN_POINT('Ctrl Pts',(-27.9375391926626,18.1062776437531,20.6984118527539));
#65572=CARTESIAN_POINT('Ctrl Pts',(-28.4549053217882,17.9439937491035,20.8392569853186));
#65573=CARTESIAN_POINT('Ctrl Pts',(-28.7362089711958,17.9037322369437,20.8735807179272));
#65574=CARTESIAN_POINT('Ctrl Pts',(-29.2637910288042,17.9037322369437,20.8735807179272));
#65575=CARTESIAN_POINT('Ctrl Pts',(-29.5450946782118,17.9439937491035,20.8392569853186));
#65576=CARTESIAN_POINT('Ctrl Pts',(-30.0624608073374,18.1062776437531,20.6984118527539));
#65577=CARTESIAN_POINT('Ctrl Pts',(-30.2985320287982,18.2281408464247,20.5917392401225));
#65578=CARTESIAN_POINT('Ctrl Pts',(-30.6713162372864,18.5059934629633,20.3423953731785));
#65579=CARTESIAN_POINT('Ctrl Pts',(-30.832915628088,18.6805067132861,20.1830533656328));
#65580=CARTESIAN_POINT('Ctrl Pts',(-31.0472603475164,19.0570372826678,19.827917294343));
#65581=CARTESIAN_POINT('Ctrl Pts',(-31.1,19.2589082724023,19.6319646928578));
#65582=CARTESIAN_POINT('Ctrl Pts',(-31.1,19.4454364826301,19.4454364826301));
#65583=CARTESIAN_POINT('',(-29.,20.8735807179272,17.9037322369437));
#65584=CARTESIAN_POINT('Ctrl Pts',(-29.,20.8735807179272,17.9037322369437));
#65585=CARTESIAN_POINT('Ctrl Pts',(-28.9409243315885,20.8735807179272,17.9037322369437));
#65586=CARTESIAN_POINT('Ctrl Pts',(-28.8823185723426,20.8719561180177,17.9056270228153));
#65587=CARTESIAN_POINT('Ctrl Pts',(-28.8241875429964,20.868766419503,17.9093441853626));
#65588=CARTESIAN_POINT('Ctrl Pts',(-28.7651735233883,20.8655282705693,17.9131178103254));
#65589=CARTESIAN_POINT('Ctrl Pts',(-28.7066479020686,20.8606771585548,17.9187695517304));
#65590=CARTESIAN_POINT('Ctrl Pts',(-28.6486082424822,20.8542378533544,17.9262611346121));
#65591=CARTESIAN_POINT('Ctrl Pts',(-28.5905518731159,20.8477966942601,17.9337548743414));
#65592=CARTESIAN_POINT('Ctrl Pts',(-28.5329808778428,20.8397663253161,17.9430896171325));
#65593=CARTESIAN_POINT('Ctrl Pts',(-28.475898465847,20.8301348968028,17.954263695967));
#65594=CARTESIAN_POINT('Ctrl Pts',(-28.4194214387268,20.8206056139583,17.9653192686261));
#65595=CARTESIAN_POINT('Ctrl Pts',(-28.3634218934566,20.809508840884,17.978175580729));
#65596=CARTESIAN_POINT('Ctrl Pts',(-28.307920773518,20.7967996666906,17.9928644519354));
#65597=CARTESIAN_POINT('Ctrl Pts',(-28.2704559732151,20.7882206204714,18.0027798487244));
#65598=CARTESIAN_POINT('Ctrl Pts',(-28.233218662767,20.7789061710475,18.01353096647));
#65599=CARTESIAN_POINT('Ctrl Pts',(-28.1962227045941,20.7688345408256,18.0251355561008));
#65600=CARTESIAN_POINT('Ctrl Pts',(-28.1419909449969,20.7540707056415,18.0421465309792));
#65601=CARTESIAN_POINT('Ctrl Pts',(-28.0891325289024,20.7379131154835,18.0607204150564));
#65602=CARTESIAN_POINT('Ctrl Pts',(-28.0376128730261,20.7204071307495,18.0807817717886));
#65603=CARTESIAN_POINT('Ctrl Pts',(-27.9853278203101,20.7026410700278,18.1011411681483));
#65604=CARTESIAN_POINT('Ctrl Pts',(-27.9344207901101,20.6834860586877,18.1230327563019));
#65605=CARTESIAN_POINT('Ctrl Pts',(-27.8848692043026,20.662952907283,18.1464142890666));
#65606=CARTESIAN_POINT('Ctrl Pts',(-27.835309647837,20.6424164530025,18.1697995828855));
#65607=CARTESIAN_POINT('Ctrl Pts',(-27.7871052343873,20.6205010894759,18.1946756264686));
#65608=CARTESIAN_POINT('Ctrl Pts',(-27.7402584745463,20.5971853396141,18.2210324451026));
#65609=CARTESIAN_POINT('Ctrl Pts',(-27.6939156433813,20.5741203963182,18.2471057445187));
#65610=CARTESIAN_POINT('Ctrl Pts',(-27.6489008029551,20.5496846281942,18.2746285373045));
#65611=CARTESIAN_POINT('Ctrl Pts',(-27.6052508789822,20.5238311574231,18.3036172535751));
#65612=CARTESIAN_POINT('Ctrl Pts',(-27.5745062838357,20.505621400804,18.3240353039275));
#65613=CARTESIAN_POINT('Ctrl Pts',(-27.5444395295393,20.4867077633294,18.3451811575672));
#65614=CARTESIAN_POINT('Ctrl Pts',(-27.5150764042051,20.4670676659985,18.3670667542599));
#65615=CARTESIAN_POINT('Ctrl Pts',(-27.4739307803984,20.4395466154596,18.3977343524141));
#65616=CARTESIAN_POINT('Ctrl Pts',(-27.4348258110997,20.4110406080958,18.4293596244423));
#65617=CARTESIAN_POINT('Ctrl Pts',(-27.397693251414,20.3815788026156,18.4618845126644));
#65618=CARTESIAN_POINT('Ctrl Pts',(-27.3600131663981,20.3516825782612,18.494888985389));
#65619=CARTESIAN_POINT('Ctrl Pts',(-27.32436345212,20.3208017675861,18.5288201934746));
#65620=CARTESIAN_POINT('Ctrl Pts',(-27.2907051878983,20.2889367073675,18.5636476038707));
#65621=CARTESIAN_POINT('Ctrl Pts',(-27.2570404826908,20.257065549318,18.5984816789854));
#65622=CARTESIAN_POINT('Ctrl Pts',(-27.225367491637,20.224209272259,18.6342127921753));
#65623=CARTESIAN_POINT('Ctrl Pts',(-27.1956878552695,20.1903450809994,18.6708335250196));
#65624=CARTESIAN_POINT('Ctrl Pts',(-27.1663254278762,20.1568428222527,18.7070628640827));
#65625=CARTESIAN_POINT('Ctrl Pts',(-27.138913630464,20.1223535486345,18.7441634385671));
#65626=CARTESIAN_POINT('Ctrl Pts',(-27.1134998926827,20.0868402088014,18.7821430446352));
#65627=CARTESIAN_POINT('Ctrl Pts',(-27.0945077136319,20.0603004012924,18.810525940726));
#65628=CARTESIAN_POINT('Ctrl Pts',(-27.0766323337211,20.0331883084273,18.8394001223222));
#65629=CARTESIAN_POINT('Ctrl Pts',(-27.0599121975429,20.0054856370759,18.868771672389));
#65630=CARTESIAN_POINT('Ctrl Pts',(-27.0375591557561,19.9684501151328,18.9080383074801));
#65631=CARTESIAN_POINT('Ctrl Pts',(-27.0176337763097,19.9309625884957,18.9475518440566));
#65632=CARTESIAN_POINT('Ctrl Pts',(-27.000049650795,19.893040530158,18.9872827250967));
#65633=CARTESIAN_POINT('Ctrl Pts',(-26.9822027462842,19.8545517606461,19.0276073485451));
#65634=CARTESIAN_POINT('Ctrl Pts',(-26.9667672171665,19.8156148371944,19.0681563988552));
#65635=CARTESIAN_POINT('Ctrl Pts',(-26.9536989008189,19.7762288706783,19.1089181312319));
#65636=CARTESIAN_POINT('Ctrl Pts',(-26.9406270335039,19.7368322020733,19.1496909395251));
#65637=CARTESIAN_POINT('Ctrl Pts',(-26.9299234702477,19.6969856526238,19.1906771391979));
#65638=CARTESIAN_POINT('Ctrl Pts',(-26.9215940204688,19.6566779068226,19.2318754015355));
#65639=CARTESIAN_POINT('Ctrl Pts',(-26.9133527431819,19.6167968439941,19.2726375542201));
#65640=CARTESIAN_POINT('Ctrl Pts',(-26.9074355517788,19.5764637104953,19.3136078904466));
#65641=CARTESIAN_POINT('Ctrl Pts',(-26.9038985506748,19.5356661328462,19.354786536779));
#65642=CARTESIAN_POINT('Ctrl Pts',(-26.9013126263588,19.5058387607383,19.3848925106586));
#65643=CARTESIAN_POINT('Ctrl Pts',(-26.9,19.4757630666449,19.4151098986153));
#65644=CARTESIAN_POINT('Ctrl Pts',(-26.9,19.4454364826301,19.4454364826301));
#65645=CARTESIAN_POINT('Ctrl Pts',(-31.1,19.4454364826301,19.4454364826301));
#65646=CARTESIAN_POINT('Ctrl Pts',(-31.1,19.6319646928578,19.2589082724023));
#65647=CARTESIAN_POINT('Ctrl Pts',(-31.0472603475164,19.827917294343,19.0570372826678));
#65648=CARTESIAN_POINT('Ctrl Pts',(-30.832915628088,20.1830533656328,18.6805067132861));
#65649=CARTESIAN_POINT('Ctrl Pts',(-30.6713162372864,20.3423953731785,18.5059934629633));
#65650=CARTESIAN_POINT('Ctrl Pts',(-30.2985320287982,20.5917392401225,18.2281408464247));
#65651=CARTESIAN_POINT('Ctrl Pts',(-30.0624608073374,20.6984118527539,18.1062776437531));
#65652=CARTESIAN_POINT('Ctrl Pts',(-29.5450946782118,20.8392569853186,17.9439937491035));
#65653=CARTESIAN_POINT('Ctrl Pts',(-29.2637910288042,20.8735807179272,17.9037322369437));
#65654=CARTESIAN_POINT('Ctrl Pts',(-29.,20.8735807179272,17.9037322369437));
#65655=CARTESIAN_POINT('Origin',(-24.,6.47002704781655,2.22738636077798));
#65656=CARTESIAN_POINT('',(-24.,10.8187337521138,6.57609306507525));
#65657=CARTESIAN_POINT('Origin',(-24.,2.22738636069727,6.47002704789727));
#65658=CARTESIAN_POINT('',(-24.,6.57609306499454,10.8187337521945));
#65659=CARTESIAN_POINT('Origin',(-24.,8.69741340855418,8.69741340863489));
#65660=CARTESIAN_POINT('Origin',(-1.,-15.9099025767,15.9099025767));
#65661=CARTESIAN_POINT('',(7.,-8.07884944143965,26.2865401242261));
#65662=CARTESIAN_POINT('',(7.,-2.97860517091918,17.244648771018));
#65663=CARTESIAN_POINT('Origin',(7.,-15.9099025767,15.9099025767));
#65664=CARTESIAN_POINT('',(-1.,-8.07884944143965,26.2865401242261));
#65665=CARTESIAN_POINT('',(-1.,-2.97860517091918,17.244648771018));
#65666=CARTESIAN_POINT('Origin',(-1.,15.9099025767,15.9099025767));
#65667=CARTESIAN_POINT('',(7.,26.2865401242261,8.07884944143965));
#65668=CARTESIAN_POINT('',(7.,17.244648771018,2.97860517091918));
#65669=CARTESIAN_POINT('Origin',(7.,15.9099025767,15.9099025767));
#65670=CARTESIAN_POINT('',(-1.,26.2865401242261,8.07884944143965));
#65671=CARTESIAN_POINT('',(-1.,17.244648771018,2.97860517091918));
#65672=CARTESIAN_POINT('Origin',(-1.,15.9099025767,-15.9099025767));
#65673=CARTESIAN_POINT('',(7.,26.2865401242261,-8.07884944143965));
#65674=CARTESIAN_POINT('',(-1.,26.2865401242261,-8.07884944143965));
#65675=CARTESIAN_POINT('',(7.,17.244648771018,-2.97860517091918));
#65676=CARTESIAN_POINT('Origin',(7.,15.9099025767,-15.9099025767));
#65677=CARTESIAN_POINT('',(-1.,17.244648771018,-2.97860517091918));
#65678=CARTESIAN_POINT('Origin',(-1.,0.,0.));
#65679=CARTESIAN_POINT('',(7.,2.97860517091918,17.244648771018));
#65680=CARTESIAN_POINT('Origin',(7.,0.,0.));
#65681=CARTESIAN_POINT('',(-1.,2.97860517091918,17.244648771018));
#65682=CARTESIAN_POINT('Origin',(-1.,0.,0.));
#65683=CARTESIAN_POINT('Origin',(7.,0.,0.));
#65684=CARTESIAN_POINT('Origin',(-1.,15.9099025767,15.9099025767));
#65685=CARTESIAN_POINT('',(7.,8.07884944143965,26.2865401242261));
#65686=CARTESIAN_POINT('',(-1.,8.07884944143965,26.2865401242261));
#65687=CARTESIAN_POINT('Origin',(7.,15.9099025767,15.9099025767));
#65688=CARTESIAN_POINT('Origin',(7.,0.,13.75));
#65689=CARTESIAN_POINT('Origin',(7.,0.,0.));
#65690=CARTESIAN_POINT('Origin',(7.,0.,13.75));
#65691=CARTESIAN_POINT('Origin',(7.,0.,0.));
#65692=CARTESIAN_POINT('Origin',(-15.25,0.,0.));
#65693=CARTESIAN_POINT('',(-4.3435534146,-2.1388888889,27.4166948102965));
#65694=CARTESIAN_POINT('',(-5.18767834635794,0.459060516890588,27.4961681592514));
#65695=CARTESIAN_POINT('Ctrl Pts',(-5.18767834635794,0.459060516890587,
27.4961681592514));
#65696=CARTESIAN_POINT('Ctrl Pts',(-5.24965809277248,0.414029595245434,
27.4969199701236));
#65697=CARTESIAN_POINT('Ctrl Pts',(-5.30712124170086,0.364629158505802,
27.4976316978157));
#65698=CARTESIAN_POINT('Ctrl Pts',(-5.48660165044913,0.185124728033571,
27.4996725546973));
#65699=CARTESIAN_POINT('Ctrl Pts',(-5.59711475871681,0.0236269477990792,
27.5005588966783));
#65700=CARTESIAN_POINT('Ctrl Pts',(-5.74364605565176,-0.330191593200779,
27.4985867159418));
#65701=CARTESIAN_POINT('Ctrl Pts',(-5.7796645257,-0.522511665581369,27.4956269007824));
#65702=CARTESIAN_POINT('Ctrl Pts',(-5.7796645257,-0.883231079115617,27.4864055040933));
#65703=CARTESIAN_POINT('Ctrl Pts',(-5.74357914128894,-1.07563756694651,
27.4795264541498));
#65704=CARTESIAN_POINT('Ctrl Pts',(-5.59693543031386,-1.42950329514698,
27.4633918271089));
#65705=CARTESIAN_POINT('Ctrl Pts',(-5.4863803371174,-1.5909684685238,27.4542371442706));
#65706=CARTESIAN_POINT('Ctrl Pts',(-5.2314028462211,-1.84584631737978,27.4382787767415));
#65707=CARTESIAN_POINT('Ctrl Pts',(-5.06999631183931,-1.9563112878812,27.4304254942484));
#65708=CARTESIAN_POINT('Ctrl Pts',(-4.71625542419335,-2.1028344711005,27.4195821238672));
#65709=CARTESIAN_POINT('Ctrl Pts',(-4.52391635613999,-2.1388888889,27.4166948102965));
#65710=CARTESIAN_POINT('Ctrl Pts',(-4.3435534146,-2.1388888889,27.4166948102965));
#65711=CARTESIAN_POINT('',(-5.7631397208,2.1388888889,27.4166948102965));
#65712=CARTESIAN_POINT('Origin',(-5.03051074634245,0.000272929993637497,
-3.21571077187848));
#65713=CARTESIAN_POINT('',(-4.7295794663,2.1388888889,27.4166948102965));
#65714=CARTESIAN_POINT('',(-5.24635959355,2.1388888889,27.4166948102965));
#65715=CARTESIAN_POINT('',(-4.2292347159,0.6783333333,27.491632615924));
#65716=CARTESIAN_POINT('Origin',(-3.9969811813186,0.000362414293276214,
-3.21399783711568));
#65717=CARTESIAN_POINT('',(-3.7202200813,0.6783333333,27.491632615924));
#65718=CARTESIAN_POINT('',(-3.9747273986,0.6783333333,27.491632615924));
#65719=CARTESIAN_POINT('',(-3.7202200813,2.1388888889,27.4166948102965));
#65720=CARTESIAN_POINT('Origin',(-3.7202200813,0.,0.));
#65721=CARTESIAN_POINT('',(-2.7424423035,2.1388888889,27.4166948102965));
#65722=CARTESIAN_POINT('',(-3.2313311924,2.1388888889,27.4166948102965));
#65723=CARTESIAN_POINT('',(-2.7424423035,-2.1388888889,27.4166948102965));
#65724=CARTESIAN_POINT('Origin',(-2.7424423035,0.,0.));
#65725=CARTESIAN_POINT('',(-3.54299785905,-2.1388888889,27.4166948102965));
#65726=CARTESIAN_POINT('',(-1.4888888889,-1.1611111111,27.4754767199348));
#65727=CARTESIAN_POINT('',(-1.4888888889,2.1388888889,27.4166948102965));
#65728=CARTESIAN_POINT('Origin',(-1.4888888889,0.,0.));
#65729=CARTESIAN_POINT('',(-0.5111111111,2.1388888889,27.4166948102965));
#65730=CARTESIAN_POINT('',(-1.,2.1388888889,27.4166948102965));
#65731=CARTESIAN_POINT('',(-0.5111111111,-1.1611111111,27.4754767199348));
#65732=CARTESIAN_POINT('Origin',(-0.5111111111,0.,0.));
#65733=CARTESIAN_POINT('',(0.5277777778,-1.1611111111,27.4754767199348));
#65734=CARTESIAN_POINT('',(0.00833333335000042,-1.1611111111,27.4754767199348));
#65735=CARTESIAN_POINT('',(0.5277777778,-2.1388888889,27.4166948102965));
#65736=CARTESIAN_POINT('Origin',(0.527777777800001,0.,0.));
#65737=CARTESIAN_POINT('',(-2.5277777778,-2.1388888889,27.4166948102965));
#65738=CARTESIAN_POINT('',(-1.,-2.1388888889,27.4166948102965));
#65739=CARTESIAN_POINT('',(-2.5277777778,-1.1611111111,27.4754767199348));
#65740=CARTESIAN_POINT('Origin',(-2.5277777778,0.,0.));
#65741=CARTESIAN_POINT('',(-2.00833333335,-1.1611111111,27.4754767199348));
#65742=CARTESIAN_POINT('',(3.7631397208,2.75,27.362154520432));
#65743=CARTESIAN_POINT('',(1.8075841652,2.75,27.362154520432));
#65744=CARTESIAN_POINT('',(2.785361943,2.75,27.362154520432));
#65745=CARTESIAN_POINT('',(-1.,4.3709594736,27.150409081267));
#65746=CARTESIAN_POINT('Origin',(6.57072389467804,-5.08186381864562E-9,
-3.39134897942017E-8));
#65747=CARTESIAN_POINT('',(-3.8075841652,2.75,27.362154520432));
#65748=CARTESIAN_POINT('Origin',(-8.57072394033692,-3.14535625323131E-8,
-2.40405939599952E-7));
#65749=CARTESIAN_POINT('',(-5.7631397208,2.75,27.362154520432));
#65750=CARTESIAN_POINT('',(-4.785361943,2.75,27.362154520432));
#65751=CARTESIAN_POINT('',(-1.,5.5,26.944387170615));
#65752=CARTESIAN_POINT('Origin',(-10.5262794172666,1.40492439903994E-8,
9.1254430678589E-8));
#65753=CARTESIAN_POINT('Origin',(8.52627943337224,4.74967842833962E-9,2.95255420112994E-8));
#65754=CARTESIAN_POINT('',(1.9747474276,-0.2016666667,27.4992605456136));
#65755=CARTESIAN_POINT('',(0.5561396937,2.1388888889,27.4166948102965));
#65756=CARTESIAN_POINT('Origin',(1.85251751839491,0.,0.));
#65757=CARTESIAN_POINT('',(1.6994942043,2.1388888889,27.4166948102965));
#65758=CARTESIAN_POINT('',(1.127816949,2.1388888889,27.4166948102965));
#65759=CARTESIAN_POINT('',(2.785361943,0.3473197978,27.4978066208572));
#65760=CARTESIAN_POINT('Origin',(2.9955115927225,0.000594682442375816,-10.0686161186405));
#65761=CARTESIAN_POINT('',(2.785361943,2.1388888889,27.4166948102965));
#65762=CARTESIAN_POINT('Origin',(2.785361943,0.,0.));
#65763=CARTESIAN_POINT('',(3.7631397208,2.1388888889,27.4166948102965));
#65764=CARTESIAN_POINT('',(3.2742508319,2.1388888889,27.4166948102965));
#65765=CARTESIAN_POINT('',(3.7631397208,-2.1388888889,27.4166948102965));
#65766=CARTESIAN_POINT('Origin',(3.7631397208,0.,0.));
#65767=CARTESIAN_POINT('',(2.785361943,-2.1388888889,27.4166948102965));
#65768=CARTESIAN_POINT('',(3.2742508319,-2.1388888889,27.4166948102965));
#65769=CARTESIAN_POINT('',(2.785361943,-0.7484330612,27.4898135307045));
#65770=CARTESIAN_POINT('Origin',(2.785361943,0.,0.));
#65771=CARTESIAN_POINT('',(1.8474876449,-2.1388888889,27.4166948102965));
#65772=CARTESIAN_POINT('Origin',(3.28939526747748,-0.001172927507095,-12.4577275280589));
#65773=CARTESIAN_POINT('',(0.6680745397,-2.1388888889,27.4166948102965));
#65774=CARTESIAN_POINT('',(1.2577810923,-2.1388888889,27.4166948102965));
#65775=CARTESIAN_POINT('Origin',(2.11077331185338,0.,0.));
#65776=CARTESIAN_POINT('',(-1.,-4.3709594736,27.150409081267));
#65777=CARTESIAN_POINT('',(1.8075841652,-2.75,27.362154520432));
#65778=CARTESIAN_POINT('Origin',(6.57072389476503,5.14153497555014E-9,-3.42402284303489E-8));
#65779=CARTESIAN_POINT('',(3.7631397208,-2.75,27.362154520432));
#65780=CARTESIAN_POINT('',(2.785361943,-2.75,27.362154520432));
#65781=CARTESIAN_POINT('',(-1.,-5.5,26.944387170615));
#65782=CARTESIAN_POINT('Origin',(8.5262794280497,-7.82302223001352E-9,5.00813346349105E-8));
#65783=CARTESIAN_POINT('',(-5.7631397208,-2.75,27.362154520432));
#65784=CARTESIAN_POINT('Origin',(-10.5262794294935,-6.98918367625367E-9,
4.45900916190567E-8));
#65785=CARTESIAN_POINT('',(-3.8075841652,-2.75,27.362154520432));
#65786=CARTESIAN_POINT('',(-4.785361943,-2.75,27.362154520432));
#65787=CARTESIAN_POINT('Origin',(-8.57072394746809,3.55609436342164E-8,
-2.70109778988115E-7));
#65788=CARTESIAN_POINT('Origin',(-1.,0.,0.));
#65789=CARTESIAN_POINT('',(-1.4888888889,2.1388888889,26.9151473026053));
#65790=CARTESIAN_POINT('',(-1.4888888889,-1.1611111111,26.9750221684372));
#65791=CARTESIAN_POINT('Origin',(-1.4888888889,0.,0.));
#65792=CARTESIAN_POINT('',(-2.5277777778,-1.1611111111,26.9750221684372));
#65793=CARTESIAN_POINT('',(-2.00833333335,-1.1611111111,26.9750221684372));
#65794=CARTESIAN_POINT('',(-2.5277777778,-2.1388888889,26.9151473026053));
#65795=CARTESIAN_POINT('Origin',(-2.5277777778,0.,0.));
#65796=CARTESIAN_POINT('',(0.5277777778,-2.1388888889,26.9151473026053));
#65797=CARTESIAN_POINT('',(-1.,-2.1388888889,26.9151473026053));
#65798=CARTESIAN_POINT('',(0.5277777778,-1.1611111111,26.9750221684372));
#65799=CARTESIAN_POINT('Origin',(0.5277777778,0.,0.));
#65800=CARTESIAN_POINT('',(-0.5111111111,-1.1611111111,26.9750221684372));
#65801=CARTESIAN_POINT('',(0.00833333334999997,-1.1611111111,26.9750221684372));
#65802=CARTESIAN_POINT('',(-0.5111111111,2.1388888889,26.9151473026053));
#65803=CARTESIAN_POINT('Origin',(-0.5111111111,0.,0.));
#65804=CARTESIAN_POINT('',(-1.,2.1388888889,26.9151473026053));
#65805=CARTESIAN_POINT('Origin',(-0.5111111111,0.4888888889,0.));
#65806=CARTESIAN_POINT('',(-0.5111111111,2.1388888889,0.));
#65807=CARTESIAN_POINT('',(-0.5111111111,-1.1611111111,0.));
#65808=CARTESIAN_POINT('Origin',(-1.,2.1388888889,0.));
#65809=CARTESIAN_POINT('',(-1.4888888889,2.1388888889,0.));
#65810=CARTESIAN_POINT('Origin',(0.00833333334999997,-1.1611111111,0.));
#65811=CARTESIAN_POINT('',(0.5277777778,-1.1611111111,0.));
#65812=CARTESIAN_POINT('Origin',(0.5277777778,-1.65,0.));
#65813=CARTESIAN_POINT('',(0.5277777778,-2.1388888889,0.));
#65814=CARTESIAN_POINT('Origin',(-1.,-2.1388888889,0.));
#65815=CARTESIAN_POINT('',(-2.5277777778,-2.1388888889,0.));
#65816=CARTESIAN_POINT('Origin',(-2.5277777778,-1.65,0.));
#65817=CARTESIAN_POINT('',(-2.5277777778,-1.1611111111,0.));
#65818=CARTESIAN_POINT('Origin',(-2.00833333335,-1.1611111111,0.));
#65819=CARTESIAN_POINT('',(-1.4888888889,-1.1611111111,0.));
#65820=CARTESIAN_POINT('Origin',(-1.4888888889,0.4888888889,0.));
#65821=CARTESIAN_POINT('Origin',(2.24242807365,1.24310434335,0.));
#65822=CARTESIAN_POINT('',(1.6994942043,2.1388888889,26.9151473026053));
#65823=CARTESIAN_POINT('',(1.6994942043,2.1388888889,0.));
#65824=CARTESIAN_POINT('',(2.785361943,0.3473197978,26.9977659993944));
#65825=CARTESIAN_POINT('Origin',(2.99587202900024,0.,0.));
#65826=CARTESIAN_POINT('',(2.785361943,0.3473197978,0.));
#65827=CARTESIAN_POINT('Origin',(1.127816949,2.1388888889,0.));
#65828=CARTESIAN_POINT('',(0.5561396937,2.1388888889,26.9151473026053));
#65829=CARTESIAN_POINT('',(0.5561396937,2.1388888889,0.));
#65830=CARTESIAN_POINT('',(1.127816949,2.1388888889,26.9151473026053));
#65831=CARTESIAN_POINT('Origin',(1.26544356065,0.9686111111,0.));
#65832=CARTESIAN_POINT('',(1.9747474276,-0.2016666667,26.9992468516354));
#65833=CARTESIAN_POINT('',(1.9747474276,-0.2016666667,0.));
#65834=CARTESIAN_POINT('Origin',(1.85251751839491,0.,0.));
#65835=CARTESIAN_POINT('Origin',(1.2577810923,-2.1388888889,0.));
#65836=CARTESIAN_POINT('',(1.8474876449,-2.1388888889,26.9151473026053));
#65837=CARTESIAN_POINT('',(1.8474876449,-2.1388888889,0.));
#65838=CARTESIAN_POINT('',(0.6680745397,-2.1388888889,26.9151473026053));
#65839=CARTESIAN_POINT('',(1.2577810923,-2.1388888889,26.9151473026053));
#65840=CARTESIAN_POINT('',(0.6680745397,-2.1388888889,0.));
#65841=CARTESIAN_POINT('Origin',(2.31642479395,-1.44366097505,0.));
#65842=CARTESIAN_POINT('',(2.785361943,-0.7484330612,26.9896248205288));
#65843=CARTESIAN_POINT('',(2.785361943,-0.7484330612,0.));
#65844=CARTESIAN_POINT('Origin',(3.289365669055,-0.00121680896187332,-12.2292518146672));
#65845=CARTESIAN_POINT('Origin',(2.785361943,-1.44366097505,0.));
#65846=CARTESIAN_POINT('',(2.785361943,-2.1388888889,26.9151473026053));
#65847=CARTESIAN_POINT('',(2.785361943,-2.1388888889,0.));
#65848=CARTESIAN_POINT('Origin',(2.785361943,0.,0.));
#65849=CARTESIAN_POINT('Origin',(3.2742508319,-2.1388888889,0.));
#65850=CARTESIAN_POINT('',(3.7631397208,-2.1388888889,26.9151473026053));
#65851=CARTESIAN_POINT('',(3.7631397208,-2.1388888889,0.));
#65852=CARTESIAN_POINT('',(3.2742508319,-2.1388888889,26.9151473026053));
#65853=CARTESIAN_POINT('Origin',(3.7631397208,0.,0.));
#65854=CARTESIAN_POINT('',(3.7631397208,2.1388888889,26.9151473026053));
#65855=CARTESIAN_POINT('',(3.7631397208,2.1388888889,0.));
#65856=CARTESIAN_POINT('Origin',(3.7631397208,0.,0.));
#65857=CARTESIAN_POINT('Origin',(3.2742508319,2.1388888889,0.));
#65858=CARTESIAN_POINT('',(2.785361943,2.1388888889,26.9151473026053));
#65859=CARTESIAN_POINT('',(2.785361943,2.1388888889,0.));
#65860=CARTESIAN_POINT('',(3.2742508319,2.1388888889,26.9151473026053));
#65861=CARTESIAN_POINT('Origin',(2.785361943,1.24310434335,0.));
#65862=CARTESIAN_POINT('Origin',(2.785361943,0.,0.));
#65863=CARTESIAN_POINT('Origin',(1.32141098365,-1.1702777778,0.));
#65864=CARTESIAN_POINT('Origin',(2.11077331185338,0.,0.));
#65865=CARTESIAN_POINT('Origin',(-1.,0.,0.));
#65866=CARTESIAN_POINT('Origin',(-1.,0.,0.));
#65867=CARTESIAN_POINT('',(-1.,5.5,26.4338797757726));
#65868=CARTESIAN_POINT('',(-5.7631397208,2.75,26.8595886044444));
#65869=CARTESIAN_POINT('Origin',(-10.5262794446456,-1.76125336537325E-9,
-1.09255759994653E-8));
#65870=CARTESIAN_POINT('',(-3.8075841652,2.75,26.8595886044444));
#65871=CARTESIAN_POINT('',(-4.785361943,2.75,26.8595886044444));
#65872=CARTESIAN_POINT('',(-1.,4.3709594736,26.6438494456065));
#65873=CARTESIAN_POINT('Origin',(-8.57072391451643,-1.65472496815866E-8,
-1.22794205914545E-7));
#65874=CARTESIAN_POINT('',(1.8075841652,2.75,26.8595886044444));
#65875=CARTESIAN_POINT('Origin',(6.57072386138071,1.41313644119734E-8,1.099020696671E-7));
#65876=CARTESIAN_POINT('',(3.7631397208,2.75,26.8595886044444));
#65877=CARTESIAN_POINT('',(2.785361943,2.75,26.8595886044444));
#65878=CARTESIAN_POINT('Origin',(8.52627943983032,1.0193068611386E-9,6.87394141607456E-9));
#65879=CARTESIAN_POINT('Origin',(-2.4037920826,3.5604797368,0.));
#65880=CARTESIAN_POINT('',(-1.,4.3709594736,0.));
#65881=CARTESIAN_POINT('',(-3.8075841652,2.75,0.));
#65882=CARTESIAN_POINT('Origin',(0.4037920826,3.5604797368,0.));
#65883=CARTESIAN_POINT('',(1.8075841652,2.75,0.));
#65884=CARTESIAN_POINT('Origin',(-4.785361943,2.75,0.));
#65885=CARTESIAN_POINT('',(-5.7631397208,2.75,0.));
#65886=CARTESIAN_POINT('Origin',(-3.3815698604,4.125,0.));
#65887=CARTESIAN_POINT('',(-1.,5.5,0.));
#65888=CARTESIAN_POINT('Origin',(1.3815698604,4.125,0.));
#65889=CARTESIAN_POINT('',(3.7631397208,2.75,0.));
#65890=CARTESIAN_POINT('Origin',(2.785361943,2.75,0.));
#65891=CARTESIAN_POINT('Origin',(-4.785361943,-2.75,0.));
#65892=CARTESIAN_POINT('',(-5.7631397208,-2.75,26.8595886044444));
#65893=CARTESIAN_POINT('',(-5.7631397208,-2.75,0.));
#65894=CARTESIAN_POINT('',(-3.8075841652,-2.75,26.8595886044444));
#65895=CARTESIAN_POINT('',(-4.785361943,-2.75,26.8595886044444));
#65896=CARTESIAN_POINT('',(-3.8075841652,-2.75,0.));
#65897=CARTESIAN_POINT('Origin',(-3.3815698604,-4.125,0.));
#65898=CARTESIAN_POINT('',(-1.,-5.5,26.4338797757726));
#65899=CARTESIAN_POINT('',(-1.,-5.5,0.));
#65900=CARTESIAN_POINT('Origin',(-10.5262794408649,-4.21045975862455E-10,
2.9073410345859E-9));
#65901=CARTESIAN_POINT('Origin',(1.3815698604,-4.125,0.));
#65902=CARTESIAN_POINT('',(3.7631397208,-2.75,26.8595886044444));
#65903=CARTESIAN_POINT('',(3.7631397208,-2.75,0.));
#65904=CARTESIAN_POINT('Origin',(8.52627944157111,-1.4747092436096E-11,
2.30344632257129E-10));
#65905=CARTESIAN_POINT('Origin',(2.785361943,-2.75,0.));
#65906=CARTESIAN_POINT('',(1.8075841652,-2.75,26.8595886044444));
#65907=CARTESIAN_POINT('',(1.8075841652,-2.75,0.));
#65908=CARTESIAN_POINT('',(2.785361943,-2.75,26.8595886044444));
#65909=CARTESIAN_POINT('Origin',(-2.4037920826,-3.5604797368,0.));
#65910=CARTESIAN_POINT('',(-1.,-4.3709594736,26.6438494456065));
#65911=CARTESIAN_POINT('Origin',(-8.5707238773724,-4.8968212817968E-9,4.16328171937153E-8));
#65912=CARTESIAN_POINT('',(-1.,-4.3709594736,0.));
#65913=CARTESIAN_POINT('Origin',(0.4037920826,-3.5604797368,0.));
#65914=CARTESIAN_POINT('Origin',(6.57072379448721,-5.27513027703819E-8,
3.97860180356702E-7));
#65915=CARTESIAN_POINT('Origin',(-1.,0.,0.));
#65916=CARTESIAN_POINT('Origin',(-4.4794070911,1.4086111111,0.));
#65917=CARTESIAN_POINT('',(-4.7295794663,2.1388888889,26.9151473026053));
#65918=CARTESIAN_POINT('',(-4.7295794663,2.1388888889,0.));
#65919=CARTESIAN_POINT('',(-4.2292347159,0.6783333333,26.9914776158871));
#65920=CARTESIAN_POINT('Origin',(-3.9969858265374,0.000375974154255831,
-3.15507438280649));
#65921=CARTESIAN_POINT('',(-4.2292347159,0.6783333333,0.));
#65922=CARTESIAN_POINT('Origin',(-5.24635959355,2.1388888889,0.));
#65923=CARTESIAN_POINT('',(-5.7631397208,2.1388888889,26.9151473026053));
#65924=CARTESIAN_POINT('',(-5.7631397208,2.1388888889,0.));
#65925=CARTESIAN_POINT('',(-5.24635959355,2.1388888889,26.9151473026053));
#65926=CARTESIAN_POINT('Origin',(-5.47540903359635,1.29897470288934,0.));
#65927=CARTESIAN_POINT('',(-5.18767834635794,0.459060516890588,26.9960971890722));
#65928=CARTESIAN_POINT('',(-5.18767834635794,0.459060516890588,0.));
#65929=CARTESIAN_POINT('Origin',(-5.03051424673138,0.000283144313856232,
-3.15681890149318));
#65930=CARTESIAN_POINT('Origin',(-4.3435534146,-0.7027777778,0.));
#65931=CARTESIAN_POINT('',(-4.3435534146,-2.1388888889,26.9151473026053));
#65932=CARTESIAN_POINT('',(-4.3435534146,-2.1388888889,0.));
#65933=CARTESIAN_POINT('Ctrl Pts',(-4.3435534146,-2.1388888889,26.9151473026053));
#65934=CARTESIAN_POINT('Ctrl Pts',(-4.52391792341369,-2.1388888889,26.9151473026053));
#65935=CARTESIAN_POINT('Ctrl Pts',(-4.71625693450842,-2.10283382592968,
26.918088482717));
#65936=CARTESIAN_POINT('Ctrl Pts',(-5.06999455179236,-1.95631203649358,
26.9291336821038));
#65937=CARTESIAN_POINT('Ctrl Pts',(-5.23139805095757,-1.84584924667606,
26.9371329701837));
#65938=CARTESIAN_POINT('Ctrl Pts',(-5.48637421277749,-1.59097645605588,
26.9533878020362));
#65939=CARTESIAN_POINT('Ctrl Pts',(-5.59693050287028,-1.42951212256183,
26.9627125508631));
#65940=CARTESIAN_POINT('Ctrl Pts',(-5.74357733669248,-1.07564498446733,
26.979146778132));
#65941=CARTESIAN_POINT('Ctrl Pts',(-5.7796645257,-0.883236025485049,26.9861535121304));
#65942=CARTESIAN_POINT('Ctrl Pts',(-5.7796645257,-0.522513729514313,26.9955458651961));
#65943=CARTESIAN_POINT('Ctrl Pts',(-5.7436467578758,-0.330194423649562,
26.9985605075207));
#65944=CARTESIAN_POINT('Ctrl Pts',(-5.59711654864042,0.0236237606196166,
27.0005692486945));
#65945=CARTESIAN_POINT('Ctrl Pts',(-5.48660381528006,0.185121924893265,
26.9996665127352));
#65946=CARTESIAN_POINT('Ctrl Pts',(-5.30712307306233,0.364627587033973,
26.9975878598176));
#65947=CARTESIAN_POINT('Ctrl Pts',(-5.24965906631465,0.414028887925648,
26.9968629383849));
#65948=CARTESIAN_POINT('Ctrl Pts',(-5.18767834635794,0.459060516890587,
26.9960971890722));
#65949=CARTESIAN_POINT('Origin',(-3.54299785905,-2.1388888889,0.));
#65950=CARTESIAN_POINT('',(-2.7424423035,-2.1388888889,26.9151473026053));
#65951=CARTESIAN_POINT('',(-2.7424423035,-2.1388888889,0.));
#65952=CARTESIAN_POINT('',(-3.54299785905,-2.1388888889,26.9151473026053));
#65953=CARTESIAN_POINT('Origin',(-3.7202200813,-0.7027777778,0.));
#65954=CARTESIAN_POINT('',(-3.7202200813,-1.1061111111,26.9773334154787));
#65955=CARTESIAN_POINT('',(-3.7202200813,-1.1061111111,0.));
#65956=CARTESIAN_POINT('',(-3.7202200813,-0.2994444445,26.9983394493931));
#65957=CARTESIAN_POINT('Origin',(-3.7202200813,0.,0.));
#65958=CARTESIAN_POINT('',(-3.7202200813,-0.2994444445,0.));
#65959=CARTESIAN_POINT('Origin',(-4.03188674795,-1.1061111111,0.));
#65960=CARTESIAN_POINT('',(-4.3435534146,-1.1061111111,26.9773334154787));
#65961=CARTESIAN_POINT('',(-4.3435534146,-1.1061111111,0.));
#65962=CARTESIAN_POINT('',(-4.03188674795,-1.1061111111,26.9773334154787));
#65963=CARTESIAN_POINT('Origin',(-2.7424423035,0.,0.));
#65964=CARTESIAN_POINT('',(-2.7424423035,2.1388888889,26.9151473026053));
#65965=CARTESIAN_POINT('',(-2.7424423035,2.1388888889,0.));
#65966=CARTESIAN_POINT('Origin',(-2.7424423035,0.,0.));
#65967=CARTESIAN_POINT('Origin',(-3.2313311924,2.1388888889,0.));
#65968=CARTESIAN_POINT('',(-3.7202200813,2.1388888889,26.9151473026053));
#65969=CARTESIAN_POINT('',(-3.7202200813,2.1388888889,0.));
#65970=CARTESIAN_POINT('',(-3.2313311924,2.1388888889,26.9151473026053));
#65971=CARTESIAN_POINT('Origin',(-3.7202200813,1.4086111111,0.));
#65972=CARTESIAN_POINT('',(-3.7202200813,0.6783333333,26.9914776158871));
#65973=CARTESIAN_POINT('',(-3.7202200813,0.6783333333,0.));
#65974=CARTESIAN_POINT('Origin',(-3.7202200813,0.,0.));
#65975=CARTESIAN_POINT('Origin',(-3.9747273986,0.6783333333,0.));
#65976=CARTESIAN_POINT('',(-3.9747273986,0.6783333333,26.9914776158871));
#65977=CARTESIAN_POINT('Origin',(-4.3435534146,-0.7027777778,0.));
#65978=CARTESIAN_POINT('',(-4.3435534146,-0.2994444445,26.9983394493931));
#65979=CARTESIAN_POINT('',(-4.3435534146,-0.2994444445,0.));
#65980=CARTESIAN_POINT('Ctrl Pts',(-4.3435534146,-1.1061111111,26.9773334154787));
#65981=CARTESIAN_POINT('Ctrl Pts',(-4.39419751981262,-1.1061111111,26.9773334154787));
#65982=CARTESIAN_POINT('Ctrl Pts',(-4.44821399727505,-1.09598960220443,
26.9777543707312));
#65983=CARTESIAN_POINT('Ctrl Pts',(-4.54757547767286,-1.05483512303673,
26.9793948590167));
#65984=CARTESIAN_POINT('Ctrl Pts',(-4.59292073016298,-1.02380242963024,
26.9806062123945));
#65985=CARTESIAN_POINT('Ctrl Pts',(-4.66454409879151,-0.952194064006125,
26.9832283238713));
#65986=CARTESIAN_POINT('Ctrl Pts',(-4.69559097470685,-0.906837278676475,
26.9848127252447));
#65987=CARTESIAN_POINT('Ctrl Pts',(-4.73676234178596,-0.807455680198994,
26.9879693009873));
#65988=CARTESIAN_POINT('Ctrl Pts',(-4.7468867479,-0.753430573531451,26.989533338241));
#65989=CARTESIAN_POINT('Ctrl Pts',(-4.7468867479,-0.652140283928571,26.9921706971532));
#65990=CARTESIAN_POINT('Ctrl Pts',(-4.73676781048986,-0.598122239682042,
26.9934199350385));
#65991=CARTESIAN_POINT('Ctrl Pts',(-4.69560563233662,-0.498744499118134,
26.9954389467467));
#65992=CARTESIAN_POINT('Ctrl Pts',(-4.66456218935101,-0.453385052203247,
26.9962168650025));
#65993=CARTESIAN_POINT('Ctrl Pts',(-4.59293647859085,-0.381763401892919,
26.9973246659964));
#65994=CARTESIAN_POINT('Ctrl Pts',(-4.54758424200201,-0.350724746147987,
26.9977298257009));
#65995=CARTESIAN_POINT('Ctrl Pts',(-4.44821398195441,-0.309565263618254,
26.9982331447194));
#65996=CARTESIAN_POINT('Ctrl Pts',(-4.39419599674402,-0.2994444445,26.9983394493931));
#65997=CARTESIAN_POINT('Ctrl Pts',(-4.3435534146,-0.2994444445,26.9983394493931));
#65998=CARTESIAN_POINT('Origin',(-4.03188674795,-0.2994444445,0.));
#65999=CARTESIAN_POINT('',(-4.03188674795,-0.2994444445,26.9983394493931));
#66000=CARTESIAN_POINT('Origin',(-1.,0.,0.));
#66674=UNCERTAINTY_MEASURE_WITH_UNIT(LENGTH_MEASURE(0.01),#66722,
'DISTANCE_ACCURACY_VALUE',
'Maximum model space distance between geometric entities at asserted c
onnectivities');
#66680=UNCERTAINTY_MEASURE_WITH_UNIT(LENGTH_MEASURE(0.01),#66722,
'DISTANCE_ACCURACY_VALUE',
'Maximum model space distance between geometric entities at asserted c
onnectivities');
#66715=(
GEOMETRIC_REPRESENTATION_CONTEXT(3)
GLOBAL_UNCERTAINTY_ASSIGNED_CONTEXT((#66674))
GLOBAL_UNIT_ASSIGNED_CONTEXT((#66722,#66724,#66725))
REPRESENTATION_CONTEXT('','3D')
);
#66721=(
GEOMETRIC_REPRESENTATION_CONTEXT(3)
GLOBAL_UNCERTAINTY_ASSIGNED_CONTEXT((#66680))
GLOBAL_UNIT_ASSIGNED_CONTEXT((#66722,#66724,#66725))
REPRESENTATION_CONTEXT('','3D')
);
#66722=(
LENGTH_UNIT()
NAMED_UNIT(*)
SI_UNIT(.MILLI.,.METRE.)
);
#66724=(
NAMED_UNIT(*)
PLANE_ANGLE_UNIT()
SI_UNIT($,.RADIAN.)
);
#66725=(
NAMED_UNIT(*)
SI_UNIT($,.STERADIAN.)
SOLID_ANGLE_UNIT()
);
#66760=SHAPE_DEFINITION_REPRESENTATION(#66820,#66924);
#66820=PRODUCT_DEFINITION_SHAPE('',$,#66965);
#66924=SHAPE_REPRESENTATION('',(#28266),#66715);
#66930=PRODUCT_DEFINITION_CONTEXT('part definition',#67052,'design');
#66965=PRODUCT_DEFINITION('Coupling Hub 1','Coupling Hub 1',#67005,#66930);
#67005=PRODUCT_DEFINITION_FORMATION('',$,#67088);
#67052=APPLICATION_CONTEXT(
'Core Data for Automotive Mechanical Design Process');
#67053=PRODUCT_CONTEXT('part definition',#67052,'mechanical');
#67088=PRODUCT('Coupling Hub 1','Coupling Hub 1',$,(#67053));
#67095=PRESENTATION_STYLE_ASSIGNMENT((#67097));
#67097=SURFACE_STYLE_USAGE(.BOTH.,#67099);
#67099=SURFACE_SIDE_STYLE('',(#67101));
#67101=SURFACE_STYLE_FILL_AREA(#67103);
#67103=FILL_AREA_STYLE('Opaque(202,209,238)',(#67105));
#67105=FILL_AREA_STYLE_COLOUR('Opaque(202,209,238)',#67107);
#67107=COLOUR_RGB('Opaque(202,209,238)',0.792156862745098,0.819607843137255,
0.933333333333333);
ENDSEC;
END-ISO-10303-21;
